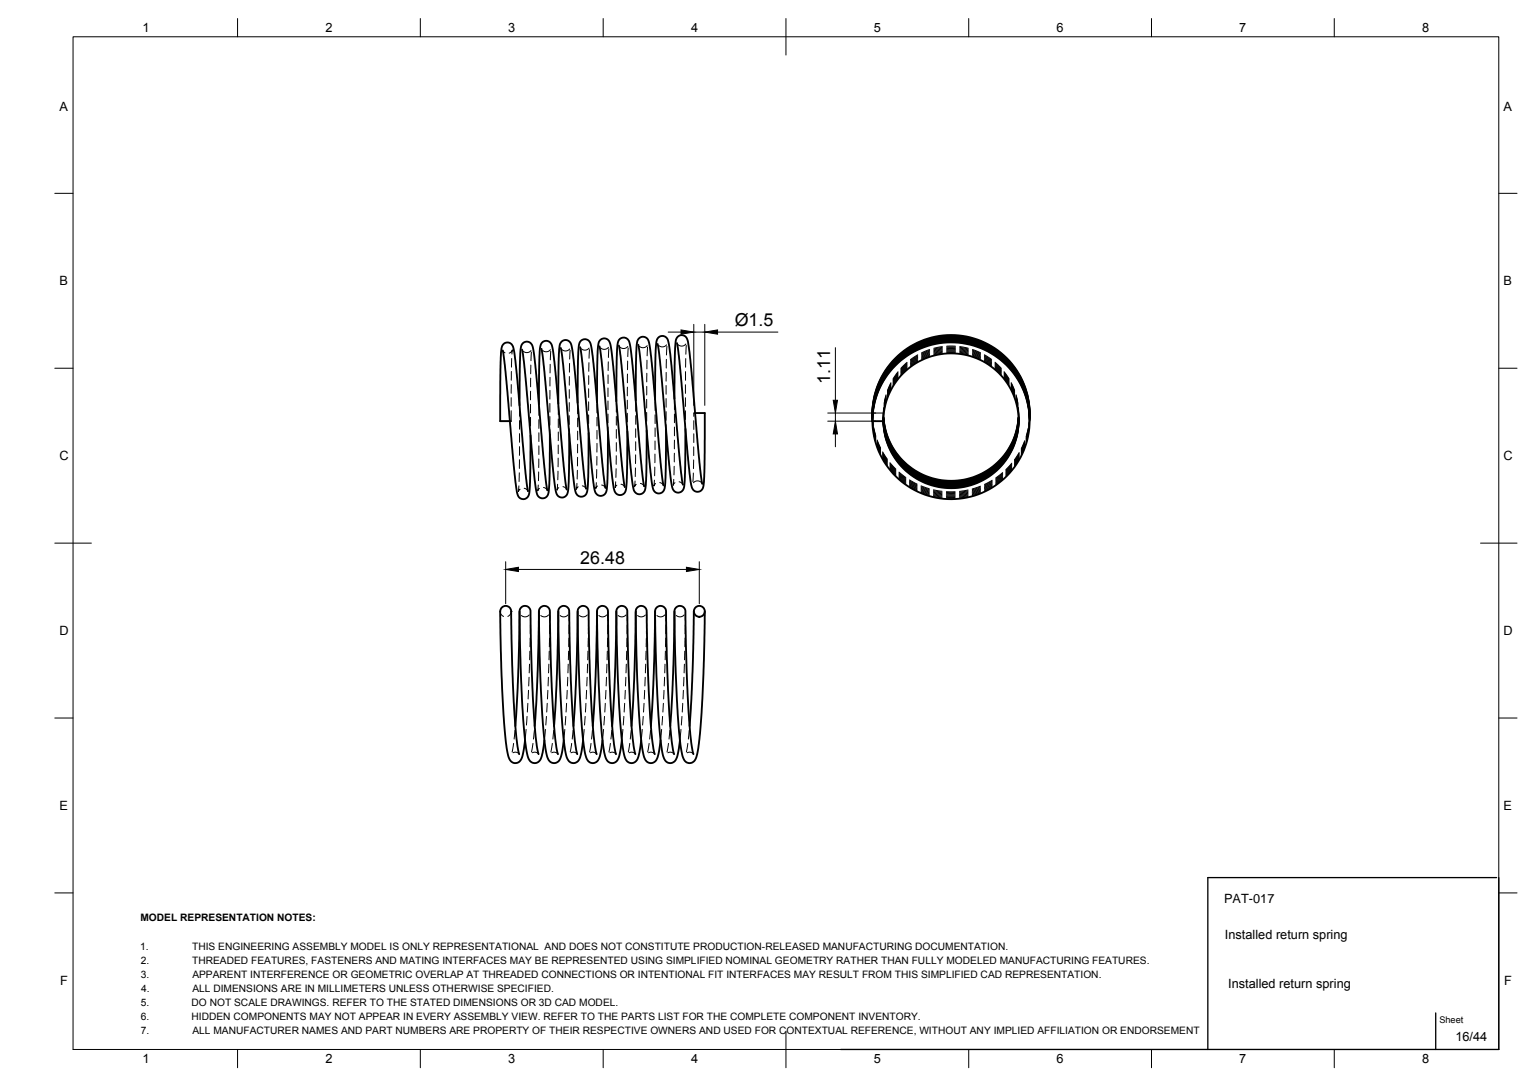
ISO-10303-21;
HEADER;
/* Generated by software containing ST-Developer
 * from STEP Tools, Inc. (www.steptools.com) 
 */

FILE_DESCRIPTION(
/* description */ ('Cam-and-follower valve demonstrator'),
/* implementation_level */ '2;1');

FILE_NAME(
/* name */ 'Installed return spring.step',
/* time_stamp */ '2026-10-28T03:25:17-07:00',
/* author */ (''),
/* organization */ (''),
/* preprocessor_version */ 'ST-DEVELOPER v20.2',
/* originating_system */ 'Autodesk Translation Framework v15.17.0.0',
/* authorisation */ '');

FILE_SCHEMA (('AUTOMOTIVE_DESIGN { 1 0 10303 214 3 1 1 }'));
ENDSEC;

DATA;
#10=MECHANICAL_DESIGN_GEOMETRIC_PRESENTATION_REPRESENTATION('',(#423),#12896);
#324=B_SPLINE_CURVE_WITH_KNOTS('',3,(#11366,#11367,#11368,#11369,#11370,
#11371,#11372,#11373,#11374,#11375,#11376,#11377,#11378,#11379,#11380,#11381,
#11382,#11383,#11384,#11385,#11386,#11387,#11388,#11389,#11390,#11391,#11392,
#11393,#11394,#11395,#11396,#11397,#11398,#11399,#11400,#11401,#11402,#11403,
#11404,#11405,#11406,#11407,#11408,#11409,#11410,#11411,#11412,#11413,#11414,
#11415,#11416,#11417,#11418,#11419,#11420,#11421,#11422,#11423,#11424,#11425,
#11426,#11427,#11428,#11429,#11430,#11431,#11432,#11433,#11434,#11435,#11436,
#11437,#11438,#11439,#11440,#11441,#11442,#11443,#11444,#11445,#11446,#11447,
#11448,#11449,#11450,#11451,#11452,#11453,#11454,#11455,#11456,#11457,#11458,
#11459,#11460,#11461,#11462,#11463,#11464,#11465,#11466,#11467,#11468,#11469,
#11470,#11471,#11472,#11473,#11474,#11475,#11476,#11477,#11478,#11479,#11480,
#11481,#11482,#11483,#11484,#11485,#11486,#11487,#11488,#11489),
 .UNSPECIFIED.,.F.,.F.,(4,1,1,1,1,1,1,1,1,1,1,1,1,1,1,1,1,1,1,1,1,1,1,1,
1,1,1,1,1,1,1,1,1,1,1,1,1,1,1,1,1,1,1,1,1,1,1,1,1,1,1,1,1,1,1,1,1,1,1,1,
1,1,1,1,1,1,1,1,1,1,1,1,1,1,1,1,1,1,1,1,1,1,1,1,1,1,1,1,1,1,1,1,1,1,1,1,
1,1,1,1,1,1,1,1,1,1,1,1,1,1,1,1,1,1,1,1,1,1,1,1,1,4),(0.,0.00892857142857143,
0.0178571428571429,0.0267857142857143,0.0357142857142857,0.0446428571428571,
0.0535714285714286,0.0625,0.0714285714285714,0.0803571428571428,0.0892857142857143,
0.0982142857142857,0.107142857142857,0.116071428571429,0.125,0.133928571428571,
0.142857142857143,0.150793650793651,0.158730158730159,0.166666666666667,
0.174603174603175,0.182539682539683,0.19047619047619,0.202380952380952,
0.214285714285714,0.222222222222222,0.23015873015873,0.238095238095238,
0.244047619047619,0.25,0.255952380952381,0.261904761904762,0.273809523809524,
0.285714285714286,0.297619047619048,0.30952380952381,0.321428571428571,
0.333333333333333,0.341269841269841,0.349206349206349,0.357142857142857,
0.365079365079365,0.373015873015873,0.375,0.376984126984127,0.380952380952381,
0.386904761904762,0.392857142857143,0.404761904761905,0.416666666666667,
0.428571428571429,0.4375,0.446428571428571,0.455357142857143,0.464285714285714,
0.468253968253968,0.476190476190476,0.482142857142857,0.488095238095238,
0.494047619047619,0.5,0.508928571428571,0.517857142857143,0.526785714285714,
0.535714285714286,0.544642857142857,0.553571428571429,0.5625,0.571428571428571,
0.580357142857143,0.589285714285714,0.598214285714286,0.607142857142857,
0.616071428571429,0.625,0.633928571428571,0.642857142857143,0.650793650793651,
0.658730158730159,0.666666666666667,0.672619047619048,0.678571428571428,
0.69047619047619,0.696428571428571,0.702380952380952,0.714285714285714,
0.726190476190476,0.732142857142857,0.738095238095238,0.746031746031746,
0.753968253968254,0.761904761904762,0.76984126984127,0.777777777777778,
0.785714285714286,0.787946428571428,0.790178571428571,0.794642857142857,
0.803571428571428,0.808035714285714,0.8125,0.821428571428571,0.830357142857143,
0.839285714285714,0.848214285714286,0.857142857142857,0.866071428571429,
0.875,0.883928571428571,0.892857142857143,0.901785714285714,0.910714285714286,
0.919642857142857,0.928571428571429,0.9375,0.946428571428571,0.955357142857143,
0.964285714285714,0.973214285714286,0.982142857142857,0.991071428571429,
1.),.UNSPECIFIED.);
#339=B_SPLINE_SURFACE_WITH_KNOTS('',3,3,((#10123,#10124,#10125,#10126,#10127,
#10128,#10129,#10130,#10131,#10132,#10133,#10134,#10135,#10136,#10137,#10138,
#10139,#10140,#10141,#10142,#10143,#10144,#10145,#10146,#10147,#10148,#10149,
#10150,#10151,#10152,#10153,#10154,#10155,#10156,#10157,#10158,#10159,#10160,
#10161,#10162,#10163,#10164,#10165,#10166,#10167,#10168,#10169,#10170,#10171,
#10172,#10173,#10174,#10175,#10176,#10177,#10178,#10179,#10180,#10181,#10182,
#10183,#10184,#10185,#10186,#10187,#10188,#10189,#10190,#10191,#10192,#10193,
#10194,#10195,#10196,#10197,#10198,#10199,#10200,#10201,#10202,#10203,#10204,
#10205,#10206,#10207,#10208,#10209,#10210,#10211,#10212,#10213,#10214,#10215,
#10216,#10217,#10218,#10219,#10220,#10221,#10222,#10223,#10224,#10225,#10226,
#10227,#10228,#10229,#10230,#10231,#10232,#10233,#10234,#10235,#10236,#10237,
#10238,#10239,#10240,#10241,#10242,#10243,#10244,#10245,#10246),(#10247,
#10248,#10249,#10250,#10251,#10252,#10253,#10254,#10255,#10256,#10257,#10258,
#10259,#10260,#10261,#10262,#10263,#10264,#10265,#10266,#10267,#10268,#10269,
#10270,#10271,#10272,#10273,#10274,#10275,#10276,#10277,#10278,#10279,#10280,
#10281,#10282,#10283,#10284,#10285,#10286,#10287,#10288,#10289,#10290,#10291,
#10292,#10293,#10294,#10295,#10296,#10297,#10298,#10299,#10300,#10301,#10302,
#10303,#10304,#10305,#10306,#10307,#10308,#10309,#10310,#10311,#10312,#10313,
#10314,#10315,#10316,#10317,#10318,#10319,#10320,#10321,#10322,#10323,#10324,
#10325,#10326,#10327,#10328,#10329,#10330,#10331,#10332,#10333,#10334,#10335,
#10336,#10337,#10338,#10339,#10340,#10341,#10342,#10343,#10344,#10345,#10346,
#10347,#10348,#10349,#10350,#10351,#10352,#10353,#10354,#10355,#10356,#10357,
#10358,#10359,#10360,#10361,#10362,#10363,#10364,#10365,#10366,#10367,#10368,
#10369,#10370),(#10371,#10372,#10373,#10374,#10375,#10376,#10377,#10378,
#10379,#10380,#10381,#10382,#10383,#10384,#10385,#10386,#10387,#10388,#10389,
#10390,#10391,#10392,#10393,#10394,#10395,#10396,#10397,#10398,#10399,#10400,
#10401,#10402,#10403,#10404,#10405,#10406,#10407,#10408,#10409,#10410,#10411,
#10412,#10413,#10414,#10415,#10416,#10417,#10418,#10419,#10420,#10421,#10422,
#10423,#10424,#10425,#10426,#10427,#10428,#10429,#10430,#10431,#10432,#10433,
#10434,#10435,#10436,#10437,#10438,#10439,#10440,#10441,#10442,#10443,#10444,
#10445,#10446,#10447,#10448,#10449,#10450,#10451,#10452,#10453,#10454,#10455,
#10456,#10457,#10458,#10459,#10460,#10461,#10462,#10463,#10464,#10465,#10466,
#10467,#10468,#10469,#10470,#10471,#10472,#10473,#10474,#10475,#10476,#10477,
#10478,#10479,#10480,#10481,#10482,#10483,#10484,#10485,#10486,#10487,#10488,
#10489,#10490,#10491,#10492,#10493,#10494),(#10495,#10496,#10497,#10498,
#10499,#10500,#10501,#10502,#10503,#10504,#10505,#10506,#10507,#10508,#10509,
#10510,#10511,#10512,#10513,#10514,#10515,#10516,#10517,#10518,#10519,#10520,
#10521,#10522,#10523,#10524,#10525,#10526,#10527,#10528,#10529,#10530,#10531,
#10532,#10533,#10534,#10535,#10536,#10537,#10538,#10539,#10540,#10541,#10542,
#10543,#10544,#10545,#10546,#10547,#10548,#10549,#10550,#10551,#10552,#10553,
#10554,#10555,#10556,#10557,#10558,#10559,#10560,#10561,#10562,#10563,#10564,
#10565,#10566,#10567,#10568,#10569,#10570,#10571,#10572,#10573,#10574,#10575,
#10576,#10577,#10578,#10579,#10580,#10581,#10582,#10583,#10584,#10585,#10586,
#10587,#10588,#10589,#10590,#10591,#10592,#10593,#10594,#10595,#10596,#10597,
#10598,#10599,#10600,#10601,#10602,#10603,#10604,#10605,#10606,#10607,#10608,
#10609,#10610,#10611,#10612,#10613,#10614,#10615,#10616,#10617,#10618),
(#10619,#10620,#10621,#10622,#10623,#10624,#10625,#10626,#10627,#10628,
#10629,#10630,#10631,#10632,#10633,#10634,#10635,#10636,#10637,#10638,#10639,
#10640,#10641,#10642,#10643,#10644,#10645,#10646,#10647,#10648,#10649,#10650,
#10651,#10652,#10653,#10654,#10655,#10656,#10657,#10658,#10659,#10660,#10661,
#10662,#10663,#10664,#10665,#10666,#10667,#10668,#10669,#10670,#10671,#10672,
#10673,#10674,#10675,#10676,#10677,#10678,#10679,#10680,#10681,#10682,#10683,
#10684,#10685,#10686,#10687,#10688,#10689,#10690,#10691,#10692,#10693,#10694,
#10695,#10696,#10697,#10698,#10699,#10700,#10701,#10702,#10703,#10704,#10705,
#10706,#10707,#10708,#10709,#10710,#10711,#10712,#10713,#10714,#10715,#10716,
#10717,#10718,#10719,#10720,#10721,#10722,#10723,#10724,#10725,#10726,#10727,
#10728,#10729,#10730,#10731,#10732,#10733,#10734,#10735,#10736,#10737,#10738,
#10739,#10740,#10741,#10742),(#10743,#10744,#10745,#10746,#10747,#10748,
#10749,#10750,#10751,#10752,#10753,#10754,#10755,#10756,#10757,#10758,#10759,
#10760,#10761,#10762,#10763,#10764,#10765,#10766,#10767,#10768,#10769,#10770,
#10771,#10772,#10773,#10774,#10775,#10776,#10777,#10778,#10779,#10780,#10781,
#10782,#10783,#10784,#10785,#10786,#10787,#10788,#10789,#10790,#10791,#10792,
#10793,#10794,#10795,#10796,#10797,#10798,#10799,#10800,#10801,#10802,#10803,
#10804,#10805,#10806,#10807,#10808,#10809,#10810,#10811,#10812,#10813,#10814,
#10815,#10816,#10817,#10818,#10819,#10820,#10821,#10822,#10823,#10824,#10825,
#10826,#10827,#10828,#10829,#10830,#10831,#10832,#10833,#10834,#10835,#10836,
#10837,#10838,#10839,#10840,#10841,#10842,#10843,#10844,#10845,#10846,#10847,
#10848,#10849,#10850,#10851,#10852,#10853,#10854,#10855,#10856,#10857,#10858,
#10859,#10860,#10861,#10862,#10863,#10864,#10865,#10866),(#10867,#10868,
#10869,#10870,#10871,#10872,#10873,#10874,#10875,#10876,#10877,#10878,#10879,
#10880,#10881,#10882,#10883,#10884,#10885,#10886,#10887,#10888,#10889,#10890,
#10891,#10892,#10893,#10894,#10895,#10896,#10897,#10898,#10899,#10900,#10901,
#10902,#10903,#10904,#10905,#10906,#10907,#10908,#10909,#10910,#10911,#10912,
#10913,#10914,#10915,#10916,#10917,#10918,#10919,#10920,#10921,#10922,#10923,
#10924,#10925,#10926,#10927,#10928,#10929,#10930,#10931,#10932,#10933,#10934,
#10935,#10936,#10937,#10938,#10939,#10940,#10941,#10942,#10943,#10944,#10945,
#10946,#10947,#10948,#10949,#10950,#10951,#10952,#10953,#10954,#10955,#10956,
#10957,#10958,#10959,#10960,#10961,#10962,#10963,#10964,#10965,#10966,#10967,
#10968,#10969,#10970,#10971,#10972,#10973,#10974,#10975,#10976,#10977,#10978,
#10979,#10980,#10981,#10982,#10983,#10984,#10985,#10986,#10987,#10988,#10989,
#10990),(#10991,#10992,#10993,#10994,#10995,#10996,#10997,#10998,#10999,
#11000,#11001,#11002,#11003,#11004,#11005,#11006,#11007,#11008,#11009,#11010,
#11011,#11012,#11013,#11014,#11015,#11016,#11017,#11018,#11019,#11020,#11021,
#11022,#11023,#11024,#11025,#11026,#11027,#11028,#11029,#11030,#11031,#11032,
#11033,#11034,#11035,#11036,#11037,#11038,#11039,#11040,#11041,#11042,#11043,
#11044,#11045,#11046,#11047,#11048,#11049,#11050,#11051,#11052,#11053,#11054,
#11055,#11056,#11057,#11058,#11059,#11060,#11061,#11062,#11063,#11064,#11065,
#11066,#11067,#11068,#11069,#11070,#11071,#11072,#11073,#11074,#11075,#11076,
#11077,#11078,#11079,#11080,#11081,#11082,#11083,#11084,#11085,#11086,#11087,
#11088,#11089,#11090,#11091,#11092,#11093,#11094,#11095,#11096,#11097,#11098,
#11099,#11100,#11101,#11102,#11103,#11104,#11105,#11106,#11107,#11108,#11109,
#11110,#11111,#11112,#11113,#11114),(#11115,#11116,#11117,#11118,#11119,
#11120,#11121,#11122,#11123,#11124,#11125,#11126,#11127,#11128,#11129,#11130,
#11131,#11132,#11133,#11134,#11135,#11136,#11137,#11138,#11139,#11140,#11141,
#11142,#11143,#11144,#11145,#11146,#11147,#11148,#11149,#11150,#11151,#11152,
#11153,#11154,#11155,#11156,#11157,#11158,#11159,#11160,#11161,#11162,#11163,
#11164,#11165,#11166,#11167,#11168,#11169,#11170,#11171,#11172,#11173,#11174,
#11175,#11176,#11177,#11178,#11179,#11180,#11181,#11182,#11183,#11184,#11185,
#11186,#11187,#11188,#11189,#11190,#11191,#11192,#11193,#11194,#11195,#11196,
#11197,#11198,#11199,#11200,#11201,#11202,#11203,#11204,#11205,#11206,#11207,
#11208,#11209,#11210,#11211,#11212,#11213,#11214,#11215,#11216,#11217,#11218,
#11219,#11220,#11221,#11222,#11223,#11224,#11225,#11226,#11227,#11228,#11229,
#11230,#11231,#11232,#11233,#11234,#11235,#11236,#11237,#11238),(#11239,
#11240,#11241,#11242,#11243,#11244,#11245,#11246,#11247,#11248,#11249,#11250,
#11251,#11252,#11253,#11254,#11255,#11256,#11257,#11258,#11259,#11260,#11261,
#11262,#11263,#11264,#11265,#11266,#11267,#11268,#11269,#11270,#11271,#11272,
#11273,#11274,#11275,#11276,#11277,#11278,#11279,#11280,#11281,#11282,#11283,
#11284,#11285,#11286,#11287,#11288,#11289,#11290,#11291,#11292,#11293,#11294,
#11295,#11296,#11297,#11298,#11299,#11300,#11301,#11302,#11303,#11304,#11305,
#11306,#11307,#11308,#11309,#11310,#11311,#11312,#11313,#11314,#11315,#11316,
#11317,#11318,#11319,#11320,#11321,#11322,#11323,#11324,#11325,#11326,#11327,
#11328,#11329,#11330,#11331,#11332,#11333,#11334,#11335,#11336,#11337,#11338,
#11339,#11340,#11341,#11342,#11343,#11344,#11345,#11346,#11347,#11348,#11349,
#11350,#11351,#11352,#11353,#11354,#11355,#11356,#11357,#11358,#11359,#11360,
#11361,#11362)),.UNSPECIFIED.,.T.,.F.,.F.,(4,1,1,1,1,1,1,4),(4,1,1,1,1,
1,1,1,1,1,1,1,1,1,1,1,1,1,1,1,1,1,1,1,1,1,1,1,1,1,1,1,1,1,1,1,1,1,1,1,1,
1,1,1,1,1,1,1,1,1,1,1,1,1,1,1,1,1,1,1,1,1,1,1,1,1,1,1,1,1,1,1,1,1,1,1,1,
1,1,1,1,1,1,1,1,1,1,1,1,1,1,1,1,1,1,1,1,1,1,1,1,1,1,1,1,1,1,1,1,1,1,1,1,
1,1,1,1,1,1,1,1,4),(-3.14159265358979,-2.24399475256414,-1.34639685153848,
-0.448798950512828,0.448798950512828,1.34639685153848,2.24399475256414,
3.14159265358979),(0.,0.00892857142857143,0.0178571428571429,0.0267857142857143,
0.0357142857142857,0.0446428571428571,0.0535714285714286,0.0625,0.0714285714285714,
0.0803571428571428,0.0892857142857143,0.0982142857142857,0.107142857142857,
0.116071428571429,0.125,0.133928571428571,0.142857142857143,0.150793650793651,
0.158730158730159,0.166666666666667,0.174603174603175,0.182539682539683,
0.19047619047619,0.202380952380952,0.214285714285714,0.222222222222222,
0.23015873015873,0.238095238095238,0.244047619047619,0.25,0.255952380952381,
0.261904761904762,0.273809523809524,0.285714285714286,0.297619047619048,
0.30952380952381,0.321428571428571,0.333333333333333,0.341269841269841,
0.349206349206349,0.357142857142857,0.365079365079365,0.373015873015873,
0.375,0.376984126984127,0.380952380952381,0.386904761904762,0.392857142857143,
0.404761904761905,0.416666666666667,0.428571428571429,0.4375,0.446428571428571,
0.455357142857143,0.464285714285714,0.468253968253968,0.476190476190476,
0.482142857142857,0.488095238095238,0.494047619047619,0.5,0.508928571428571,
0.517857142857143,0.526785714285714,0.535714285714286,0.544642857142857,
0.553571428571429,0.5625,0.571428571428571,0.580357142857143,0.589285714285714,
0.598214285714286,0.607142857142857,0.616071428571429,0.625,0.633928571428571,
0.642857142857143,0.650793650793651,0.658730158730159,0.666666666666667,
0.672619047619048,0.678571428571428,0.69047619047619,0.696428571428571,
0.702380952380952,0.714285714285714,0.726190476190476,0.732142857142857,
0.738095238095238,0.746031746031746,0.753968253968254,0.761904761904762,
0.76984126984127,0.777777777777778,0.785714285714286,0.787946428571428,
0.790178571428571,0.794642857142857,0.803571428571428,0.808035714285714,
0.8125,0.821428571428571,0.830357142857143,0.839285714285714,0.848214285714286,
0.857142857142857,0.866071428571429,0.875,0.883928571428571,0.892857142857143,
0.901785714285714,0.910714285714286,0.919642857142857,0.928571428571429,
0.9375,0.946428571428571,0.955357142857143,0.964285714285714,0.973214285714286,
0.982142857142857,0.991071428571429,1.),.UNSPECIFIED.);
#351=SHAPE_REPRESENTATION_RELATIONSHIP('SRR','None',#13067,#387);
#387=ADVANCED_BREP_SHAPE_REPRESENTATION('',(#466),#12867);
#423=STYLED_ITEM('',(#13330),#466);
#466=MANIFOLD_SOLID_BREP('Body1',#6190);
#789=CIRCLE('',#6910,0.075);
#790=CIRCLE('',#6911,0.075);
#1239=FACE_OUTER_BOUND('',#1716,.T.);
#1240=FACE_OUTER_BOUND('',#1717,.T.);
#1241=FACE_OUTER_BOUND('',#1718,.T.);
#1716=EDGE_LOOP('',(#4749,#4750,#4751,#4752));
#1717=EDGE_LOOP('',(#4753));
#1718=EDGE_LOOP('',(#4754));
#3057=VERTEX_POINT('',#11363);
#3058=VERTEX_POINT('',#11365);
#3671=EDGE_CURVE('',#3057,#3057,#789,.T.);
#3672=EDGE_CURVE('',#3057,#3058,#324,.T.);
#3673=EDGE_CURVE('',#3058,#3058,#790,.T.);
#4749=ORIENTED_EDGE('',*,*,#3671,.T.);
#4750=ORIENTED_EDGE('',*,*,#3672,.T.);
#4751=ORIENTED_EDGE('',*,*,#3673,.F.);
#4752=ORIENTED_EDGE('',*,*,#3672,.F.);
#4753=ORIENTED_EDGE('',*,*,#3673,.T.);
#4754=ORIENTED_EDGE('',*,*,#3671,.F.);
#5676=PLANE('',#6912);
#5677=PLANE('',#6913);
#5955=ADVANCED_FACE('',(#1239),#339,.T.);
#5956=ADVANCED_FACE('',(#1240),#5676,.T.);
#5957=ADVANCED_FACE('',(#1241),#5677,.F.);
#6190=CLOSED_SHELL('',(#5955,#5956,#5957));
#6909=AXIS2_PLACEMENT_3D('',#10122,#8185,#8186);
#6910=AXIS2_PLACEMENT_3D('',#11364,#8187,#8188);
#6911=AXIS2_PLACEMENT_3D('',#11490,#8189,#8190);
#6912=AXIS2_PLACEMENT_3D('',#11491,#8191,#8192);
#6913=AXIS2_PLACEMENT_3D('',#11492,#8193,#8194);
#8185=DIRECTION('axis',(0.,0.,1.));
#8186=DIRECTION('refdir',(1.,0.,0.));
#8187=DIRECTION('center_axis',(-0.00013450227597807,0.999117050244768,0.042013114849203));
#8188=DIRECTION('ref_axis',(5.65585335115278E-6,-0.0420131144685042,0.999117059298192));
#8189=DIRECTION('center_axis',(0.000134502259908405,0.999117050228794,0.0420131152291186));
#8190=DIRECTION('ref_axis',(-0.474109261639291,0.0370548329511252,-0.879685936788131));
#8191=DIRECTION('center_axis',(0.000134502259908405,0.999117050228794,0.0420131152291186));
#8192=DIRECTION('ref_axis',(-0.474109261639291,0.0370548329511252,-0.879685936788131));
#8193=DIRECTION('center_axis',(-0.00013450227597807,0.999117050244768,0.042013114849203));
#8194=DIRECTION('ref_axis',(5.65585335115278E-6,-0.0420131144685042,0.999117059298193));
#10122=CARTESIAN_POINT('',(0.,0.,0.));
#10123=CARTESIAN_POINT('Ctrl Pts',(0.999999575810999,0.00315098358513781,
7.20006622055264));
#10124=CARTESIAN_POINT('Ctrl Pts',(0.999974319608277,0.190760468856422,
7.20795524501636));
#10125=CARTESIAN_POINT('Ctrl Pts',(0.892344234443071,0.564401735476683,
7.22374165130483));
#10126=CARTESIAN_POINT('Ctrl Pts',(0.456170863303355,0.954569139239392,
7.24746551842362));
#10127=CARTESIAN_POINT('Ctrl Pts',(-0.121643296695006,1.0527111229517,7.27123039275792));
#10128=CARTESIAN_POINT('Ctrl Pts',(-0.664174499114347,0.828146653873478,
7.29503750827097));
#10129=CARTESIAN_POINT('Ctrl Pts',(-1.00466229107333,0.348451955041142,
7.31888617441183));
#10130=CARTESIAN_POINT('Ctrl Pts',(-1.03783821085617,-0.239862803165599,
7.34277653444097));
#10131=CARTESIAN_POINT('Ctrl Pts',(-0.752436914310739,-0.756562482852077,
7.36670833282365));
#10132=CARTESIAN_POINT('Ctrl Pts',(-0.234997931414651,-1.04270891419437,
7.39068146490982));
#10133=CARTESIAN_POINT('Ctrl Pts',(0.356377432582172,-1.00964746384867,
7.41469572763747));
#10134=CARTESIAN_POINT('Ctrl Pts',(0.840341677037224,-0.666437865062604,
7.43875093208249));
#10135=CARTESIAN_POINT('Ctrl Pts',(1.06790358406505,-0.117422164195028,
7.4628468515188));
#10136=CARTESIAN_POINT('Ctrl Pts',(0.968336509361683,0.469494166098508,
7.48698324256581));
#10137=CARTESIAN_POINT('Ctrl Pts',(0.571081336399399,0.914217869413367,
7.51115983904362));
#10138=CARTESIAN_POINT('Ctrl Pts',(-0.00276942901145937,1.07968430615977,
7.53537635143244));
#10139=CARTESIAN_POINT('Ctrl Pts',(-0.577781503135752,0.914223804149117,
7.55963247041146));
#10140=CARTESIAN_POINT('Ctrl Pts',(-0.962145622562424,0.483976677731404,
7.58302803095162));
#10141=CARTESIAN_POINT('Ctrl Pts',(-1.07125753086067,-0.0562794445165808,
7.60555779623404));
#10142=CARTESIAN_POINT('Ctrl Pts',(-0.915194862614763,-0.562561634031091,
7.6272168563822));
#10143=CARTESIAN_POINT('Ctrl Pts',(-0.53551487530705,-0.932963762094015,
7.64890612590553));
#10144=CARTESIAN_POINT('Ctrl Pts',(-0.024035065806305,-1.07736876663697,
7.67062531437742));
#10145=CARTESIAN_POINT('Ctrl Pts',(0.494146757015346,-0.958466814289234,
7.69237411680017));
#10146=CARTESIAN_POINT('Ctrl Pts',(0.961479539986573,-0.548279772601945,
7.71778190065853));
#10147=CARTESIAN_POINT('Ctrl Pts',(1.12756301652098,0.172482400610549,7.74686765103336));
#10148=CARTESIAN_POINT('Ctrl Pts',(0.75611713355168,0.813684959589575,7.77601030696451));
#10149=CARTESIAN_POINT('Ctrl Pts',(0.185875815215743,1.06965010757807,7.80155082448588));
#10150=CARTESIAN_POINT('Ctrl Pts',(-0.348517058347165,1.02984652160674,
7.82347022110603));
#10151=CARTESIAN_POINT('Ctrl Pts',(-0.761949296282463,0.762592777124389,
7.84358787235736));
#10152=CARTESIAN_POINT('Ctrl Pts',(-0.996722963062006,0.388518849169714,
7.86189613571743));
#10153=CARTESIAN_POINT('Ctrl Pts',(-1.07098690831041,-0.00260829917091459,
7.87838843437341));
#10154=CARTESIAN_POINT('Ctrl Pts',(-0.99661183226746,-0.393594984460838,
7.894895410549));
#10155=CARTESIAN_POINT('Ctrl Pts',(-0.714908576434247,-0.844892296878379,
7.9169240469514));
#10156=CARTESIAN_POINT('Ctrl Pts',(-0.084422651145012,-1.14985023564212,
7.94449562780488));
#10157=CARTESIAN_POINT('Ctrl Pts',(0.721887320494981,-0.901498071462995,
7.97763725360595));
#10158=CARTESIAN_POINT('Ctrl Pts',(1.14390600676876,-0.170383526932712,
8.01083302661308));
#10159=CARTESIAN_POINT('Ctrl Pts',(0.956311918053777,0.65401391794098,8.04408130906187));
#10160=CARTESIAN_POINT('Ctrl Pts',(0.25602906697655,1.13176193513965,8.07738040653961));
#10161=CARTESIAN_POINT('Ctrl Pts',(-0.488510543500641,1.01860423556296,
8.10702323570327));
#10162=CARTESIAN_POINT('Ctrl Pts',(-0.942716248260153,0.573655629467007,
8.13299136011509));
#10163=CARTESIAN_POINT('Ctrl Pts',(-1.10358636285334,0.0534364176198665,
8.15527022722507));
#10164=CARTESIAN_POINT('Ctrl Pts',(-0.99543872479676,-0.481361877750802,
8.17756901902506));
#10165=CARTESIAN_POINT('Ctrl Pts',(-0.644826641417894,-0.899786909633448,
8.1998871769012));
#10166=CARTESIAN_POINT('Ctrl Pts',(-0.263312902512338,-1.04918995788175,
8.21663989380025));
#10167=CARTESIAN_POINT('Ctrl Pts',(0.00166665731618679,-1.0655343402046,
8.22781406534667));
#10168=CARTESIAN_POINT('Ctrl Pts',(0.178270288589001,-1.05454413855026,
8.23526501957515));
#10169=CARTESIAN_POINT('Ctrl Pts',(0.437439999691742,-0.98876491629653,
8.24644481283225));
#10170=CARTESIAN_POINT('Ctrl Pts',(0.741357296669408,-0.797196125183601,
8.26135855011107));
#10171=CARTESIAN_POINT('Ctrl Pts',(1.06427742047819,-0.363196133741635,
8.28374205636937));
#10172=CARTESIAN_POINT('Ctrl Pts',(1.1191132547847,0.345488423812591,8.31174498186711));
#10173=CARTESIAN_POINT('Ctrl Pts',(0.584140656179565,1.01596202851522,8.34538413710338));
#10174=CARTESIAN_POINT('Ctrl Pts',(-0.19096844855633,1.13165287559935,8.37625078730322));
#10175=CARTESIAN_POINT('Ctrl Pts',(-0.797411359462935,0.795301993540907,
8.40433431031039));
#10176=CARTESIAN_POINT('Ctrl Pts',(-1.0990783559073,0.250015446968417,8.4296262708737));
#10177=CARTESIAN_POINT('Ctrl Pts',(-1.06426569125542,-0.373802040240765,
8.45493410201599));
#10178=CARTESIAN_POINT('Ctrl Pts',(-0.769553388901587,-0.788092512102153,
8.47556748693345));
#10179=CARTESIAN_POINT('Ctrl Pts',(-0.367608264833719,-1.03377453912702,
8.49527086803642));
#10180=CARTESIAN_POINT('Ctrl Pts',(0.0389894662197936,-1.10568483145998,
8.51216552927169));
#10181=CARTESIAN_POINT('Ctrl Pts',(0.476842798425807,-0.987859734068039,
8.53094473644388));
#10182=CARTESIAN_POINT('Ctrl Pts',(0.805101130351003,-0.7459169684144,8.54785141982868));
#10183=CARTESIAN_POINT('Ctrl Pts',(1.02206224073455,-0.400294829517718,
8.56476322077897));
#10184=CARTESIAN_POINT('Ctrl Pts',(1.11108597940432,0.0676090739442989,
8.58449929513004));
#10185=CARTESIAN_POINT('Ctrl Pts',(0.957486327179168,0.602305552598091,
8.60706239241156));
#10186=CARTESIAN_POINT('Ctrl Pts',(0.490319176226327,1.0196961225561,8.63245514939238));
#10187=CARTESIAN_POINT('Ctrl Pts',(-0.127227772869885,1.12465246691674,
8.65785621578684));
#10188=CARTESIAN_POINT('Ctrl Pts',(-0.706252354762176,0.884861784560879,
8.6832646175365));
#10189=CARTESIAN_POINT('Ctrl Pts',(-1.06898139570907,0.373646110671472,
8.70867937640931));
#10190=CARTESIAN_POINT('Ctrl Pts',(-1.10415883703196,-0.252336062683339,
8.73409951326223));
#10191=CARTESIAN_POINT('Ctrl Pts',(-0.800834752831557,-0.801177522527246,
8.75952404569165));
#10192=CARTESIAN_POINT('Ctrl Pts',(-0.251930241323733,-1.10455619700772,
8.78495198825788));
#10193=CARTESIAN_POINT('Ctrl Pts',(0.374309533721303,-1.06939244573458,
8.81038235029736));
#10194=CARTESIAN_POINT('Ctrl Pts',(0.88588373813812,-0.706416051605379,
8.83581414648952));
#10195=CARTESIAN_POINT('Ctrl Pts',(1.12593002076033,-0.126889341474946,
8.86124638643539));
#10196=CARTESIAN_POINT('Ctrl Pts',(1.02087104515559,0.491507891337351,8.88667807898767));
#10197=CARTESIAN_POINT('Ctrl Pts',(0.602911335681679,0.959196578831539,
8.91210823370906));
#10198=CARTESIAN_POINT('Ctrl Pts',(0.000316973456126708,1.13280882473463,
8.93753586563178));
#10199=CARTESIAN_POINT('Ctrl Pts',(-0.602311983560242,0.959240722445107,
8.9629599838141));
#10200=CARTESIAN_POINT('Ctrl Pts',(-1.00436822137552,0.509038661422071,
8.98743813657581));
#10201=CARTESIAN_POINT('Ctrl Pts',(-1.11811011681427,-0.0552669144060651,
9.01097002817133));
#10202=CARTESIAN_POINT('Ctrl Pts',(-0.955644771077333,-0.583087731975911,
9.03355562561233));
#10203=CARTESIAN_POINT('Ctrl Pts',(-0.593074356957321,-0.936728146430118,
9.0542538609391));
#10204=CARTESIAN_POINT('Ctrl Pts',(-0.164731041598437,-1.08578943530602,
9.07306578079699));
#10205=CARTESIAN_POINT('Ctrl Pts',(0.380219776536112,-1.06693040182505,
9.09563491033651));
#10206=CARTESIAN_POINT('Ctrl Pts',(0.853779549938941,-0.745621203287222,
9.11819570154211));
#10207=CARTESIAN_POINT('Ctrl Pts',(1.06953462325323,-0.245092836305948,
9.14074702398398));
#10208=CARTESIAN_POINT('Ctrl Pts',(1.09185195352203,0.298202592837182,9.16329164905568));
#10209=CARTESIAN_POINT('Ctrl Pts',(0.734297058725123,0.919425032182445,
9.19145918094331));
#10210=CARTESIAN_POINT('Ctrl Pts',(0.0501860572080287,1.12913650428628,
9.21960716991184));
#10211=CARTESIAN_POINT('Ctrl Pts',(-0.47422284767955,0.986938013732599,
9.24211273100823));
#10212=CARTESIAN_POINT('Ctrl Pts',(-0.83834294439581,0.718994011703782,
9.26085993499593));
#10213=CARTESIAN_POINT('Ctrl Pts',(-1.0797140885543,0.276058653254629,9.28147192866405));
#10214=CARTESIAN_POINT('Ctrl Pts',(-1.0792869722179,-0.273490761429736,
9.30394472055128));
#10215=CARTESIAN_POINT('Ctrl Pts',(-0.816874083948392,-0.756154521252702,
9.32640385818033));
#10216=CARTESIAN_POINT('Ctrl Pts',(-0.355458797527567,-1.05362205517351,
9.34884870640624));
#10217=CARTESIAN_POINT('Ctrl Pts',(0.191577194376755,-1.09493860698716,
9.37127864639074));
#10218=CARTESIAN_POINT('Ctrl Pts',(0.571484722667441,-0.923210767165354,
9.38832293897591));
#10219=CARTESIAN_POINT('Ctrl Pts',(0.775578610165073,-0.735373724461368,
9.39999172743641));
#10220=CARTESIAN_POINT('Ctrl Pts',(0.90219668945127,-0.581077610283799,
9.40839153478326));
#10221=CARTESIAN_POINT('Ctrl Pts',(1.06423218001646,-0.268505675241936,
9.42308663622534));
#10222=CARTESIAN_POINT('Ctrl Pts',(1.08737574685665,0.14445700622961,9.43987039483926));
#10223=CARTESIAN_POINT('Ctrl Pts',(0.943512119332504,0.519555849049532,
9.45664308969273));
#10224=CARTESIAN_POINT('Ctrl Pts',(0.702595952885493,0.840663912121189,
9.47340826939813));
#10225=CARTESIAN_POINT('Ctrl Pts',(0.250731034525726,1.09066378632527,9.49435038976507));
#10226=CARTESIAN_POINT('Ctrl Pts',(-0.367646366337481,1.05577469318307,
9.51945715090945));
#10227=CARTESIAN_POINT('Ctrl Pts',(-0.872073427555176,0.697769149747224,
9.54453931621249));
#10228=CARTESIAN_POINT('Ctrl Pts',(-1.10851395153864,0.126754498956172,
9.56959609551394));
#10229=CARTESIAN_POINT('Ctrl Pts',(-1.004997965557,-0.481859237919703,9.59462670660628));
#10230=CARTESIAN_POINT('Ctrl Pts',(-0.593994937248818,-0.94163509404227,
9.61963038098806));
#10231=CARTESIAN_POINT('Ctrl Pts',(-0.0020235655980388,-1.11207375119343,
9.6446063758667));
#10232=CARTESIAN_POINT('Ctrl Pts',(0.589215999041395,-0.941636436533483,
9.66955394755264));
#10233=CARTESIAN_POINT('Ctrl Pts',(0.99867475328867,-0.483298149068583,
9.69447238340543));
#10234=CARTESIAN_POINT('Ctrl Pts',(1.10139617547556,0.121906639873499,9.71936097538517));
#10235=CARTESIAN_POINT('Ctrl Pts',(0.866669607038716,0.688301956936916,
9.74421904187644));
#10236=CARTESIAN_POINT('Ctrl Pts',(0.367204775824758,1.0425526426198,9.76904590972932));
#10237=CARTESIAN_POINT('Ctrl Pts',(-0.243395435261487,1.07672488055471,
9.79384092765142));
#10238=CARTESIAN_POINT('Ctrl Pts',(-0.777888567237211,0.781186417289152,
9.81860345995005));
#10239=CARTESIAN_POINT('Ctrl Pts',(-1.07283036518199,0.247282943918733,
9.84333289822209));
#10240=CARTESIAN_POINT('Ctrl Pts',(-1.03856704754786,-0.360866232625645,
9.86802861303319));
#10241=CARTESIAN_POINT('Ctrl Pts',(-0.686501281653619,-0.856920605922548,
9.892690097101));
#10242=CARTESIAN_POINT('Ctrl Pts',(-0.125304938207573,-1.08924443021579,
9.91731661435472));
#10243=CARTESIAN_POINT('Ctrl Pts',(0.472593334675849,-0.987703022851267,
9.94190800522239));
#10244=CARTESIAN_POINT('Ctrl Pts',(0.924078607982629,-0.583894056083662,
9.9664628819065));
#10245=CARTESIAN_POINT('Ctrl Pts',(1.03553205098759,-0.196980695813872,
9.98281022139497));
#10246=CARTESIAN_POINT('Ctrl Pts',(1.03555819462295,-0.00277911247133682,
9.99097644525911));
#10247=CARTESIAN_POINT('Ctrl Pts',(0.977559628488695,0.00314796269385491,
7.20006622055264));
#10248=CARTESIAN_POINT('Ctrl Pts',(0.977534931919559,0.186600347624405,
7.20778043793643));
#10249=CARTESIAN_POINT('Ctrl Pts',(0.872326621716519,0.551848843788545,
7.22321134603222));
#10250=CARTESIAN_POINT('Ctrl Pts',(0.445888516650333,0.933334827963534,
7.24640607517782));
#10251=CARTESIAN_POINT('Ctrl Pts',(-0.119073548305639,1.02929389999416,
7.26964128868359));
#10252=CARTESIAN_POINT('Ctrl Pts',(-0.649587147996202,0.80971547210797,
7.29292023194622));
#10253=CARTESIAN_POINT('Ctrl Pts',(-0.982569682264781,0.340608289962485,
7.31624170699604));
#10254=CARTESIAN_POINT('Ctrl Pts',(-1.01502761301115,-0.234786092628464,
7.33960648723202));
#10255=CARTESIAN_POINT('Ctrl Pts',(-0.735871175247769,-0.740204838677808,
7.36301444474564));
#10256=CARTESIAN_POINT('Ctrl Pts',(-0.229676322236327,-1.02014816093488,
7.3864658304475));
#10257=CARTESIAN_POINT('Ctrl Pts',(0.348937939981405,-0.987814457701798,
7.4099606987694));
#10258=CARTESIAN_POINT('Ctrl Pts',(0.822539330220122,-0.651972394453966,
7.43349915759815));
#10259=CARTESIAN_POINT('Ctrl Pts',(1.04527595941213,-0.114640290127698,
7.45708126355647));
#10260=CARTESIAN_POINT('Ctrl Pts',(0.947826468806296,0.459896400546727,
7.48070704898826));
#10261=CARTESIAN_POINT('Ctrl Pts',(0.55889347637454,0.895331088517642,7.50437654814852));
#10262=CARTESIAN_POINT('Ctrl Pts',(-0.00306079128538847,1.05738788811831,
7.52808969478327));
#10263=CARTESIAN_POINT('Ctrl Pts',(-0.566280527706047,0.895342454830755,
7.55184656451516));
#10264=CARTESIAN_POINT('Ctrl Pts',(-0.94285566098478,0.473846121224849,
7.57476532068617));
#10265=CARTESIAN_POINT('Ctrl Pts',(-1.0497916614659,-0.0555531181652621,
7.59684113555968));
#10266=CARTESIAN_POINT('Ctrl Pts',(-0.896848267782611,-0.551773383072111,
7.6180679179377));
#10267=CARTESIAN_POINT('Ctrl Pts',(-0.524644889084921,-0.914897925677014,
7.63932924215096));
#10268=CARTESIAN_POINT('Ctrl Pts',(-0.0231086211666074,-1.0565167949332,
7.66062527908679));
#10269=CARTESIAN_POINT('Ctrl Pts',(0.485127965286644,-0.939908247511382,
7.6819553795526));
#10270=CARTESIAN_POINT('Ctrl Pts',(0.943615377154503,-0.537522345290259,
7.70687961457021));
#10271=CARTESIAN_POINT('Ctrl Pts',(1.10664549720515,0.169763989700331,7.73541865071932));
#10272=CARTESIAN_POINT('Ctrl Pts',(0.742051547502606,0.79926014258511,7.76402418077492));
#10273=CARTESIAN_POINT('Ctrl Pts',(0.1820386242008,1.05066099789059,7.78910535841451));
#10274=CARTESIAN_POINT('Ctrl Pts',(-0.342925213792071,1.01157659627672,
7.81063708262925));
#10275=CARTESIAN_POINT('Ctrl Pts',(-0.749174696900719,0.748993162117811,
7.83040267717073));
#10276=CARTESIAN_POINT('Ctrl Pts',(-0.979935807647696,0.381329024216996,
7.84839633933116));
#10277=CARTESIAN_POINT('Ctrl Pts',(-1.05295127075641,-0.0031834724715258,
7.86460871683656));
#10278=CARTESIAN_POINT('Ctrl Pts',(-0.979823859029814,-0.387650529628831,
7.88083924305493));
#10279=CARTESIAN_POINT('Ctrl Pts',(-0.702763365403678,-0.831532214326253,
7.9025045281952));
#10280=CARTESIAN_POINT('Ctrl Pts',(-0.0824799953521556,-1.13161645631995,
7.92962705663339));
#10281=CARTESIAN_POINT('Ctrl Pts',(0.711242926121418,-0.887223370319477,
7.9622469399467));
#10282=CARTESIAN_POINT('Ctrl Pts',(1.12693381986534,-0.167219554477753,
7.99493570676171));
#10283=CARTESIAN_POINT('Ctrl Pts',(0.942170158410588,0.645122540676551,
8.02769289174508));
#10284=CARTESIAN_POINT('Ctrl Pts',(0.251833448908431,1.11619302546554,8.06051740773355));
#10285=CARTESIAN_POINT('Ctrl Pts',(-0.482576734552971,1.00466065240982,
8.08975175083041));
#10286=CARTESIAN_POINT('Ctrl Pts',(-0.930837186086348,0.565588449238039,
8.1153761207135));
#10287=CARTESIAN_POINT('Ctrl Pts',(-1.08967697962172,0.0520404847636478,
8.13736727171514));
#10288=CARTESIAN_POINT('Ctrl Pts',(-0.982903963949899,-0.476104949614679,
8.15938616711863));
#10289=CARTESIAN_POINT('Ctrl Pts',(-0.636540954845654,-0.889508172876264,
8.18143408833578));
#10290=CARTESIAN_POINT('Ctrl Pts',(-0.259505287977444,-1.03717085636039,
8.1979881155864));
#10291=CARTESIAN_POINT('Ctrl Pts',(0.00245412741644389,-1.05333143683712,
8.20903477211785));
#10292=CARTESIAN_POINT('Ctrl Pts',(0.177059177795229,-1.04246573347879,
8.21640112872543));
#10293=CARTESIAN_POINT('Ctrl Pts',(0.433327913156591,-0.977427600945312,
8.22745510314132));
#10294=CARTESIAN_POINT('Ctrl Pts',(0.73391120866048,-0.78797120607176,8.2422033360845));
#10295=CARTESIAN_POINT('Ctrl Pts',(1.05339268942341,-0.358614771787532,
8.26434632322957));
#10296=CARTESIAN_POINT('Ctrl Pts',(1.10774289737246,0.342815554655969,8.29206074311086));
#10297=CARTESIAN_POINT('Ctrl Pts',(0.578013407396415,1.00685700818336,8.32536809202379));
#10298=CARTESIAN_POINT('Ctrl Pts',(-0.190065697378914,1.12158925721513,
8.35595007218663));
#10299=CARTESIAN_POINT('Ctrl Pts',(-0.791379955781598,0.788136209353913,
8.38379141767993));
#10300=CARTESIAN_POINT('Ctrl Pts',(-1.09065818214293,0.247264712325509,
8.40887610904288));
#10301=CARTESIAN_POINT('Ctrl Pts',(-1.05615602025911,-0.371820083200091,
8.43398889502081));
#10302=CARTESIAN_POINT('Ctrl Pts',(-0.763582331280387,-0.783164528531196,
8.45447107190819));
#10303=CARTESIAN_POINT('Ctrl Pts',(-0.364356836371496,-1.02719384800769,
8.47404015218794));
#10304=CARTESIAN_POINT('Ctrl Pts',(0.0396184639487176,-1.0986608375699,
8.49082507049449));
#10305=CARTESIAN_POINT('Ctrl Pts',(0.4747993472484,-0.981570587611574,8.5094874174984));
#10306=CARTESIAN_POINT('Ctrl Pts',(0.801179445412529,-0.741029716701455,
8.52629619867346));
#10307=CARTESIAN_POINT('Ctrl Pts',(1.01695965272321,-0.397307355171047,
8.54311315644057));
#10308=CARTESIAN_POINT('Ctrl Pts',(1.10554233979669,0.0681936417011055,
8.56274660530892));
#10309=CARTESIAN_POINT('Ctrl Pts',(0.952705524054136,0.600346322280504,
8.5851983552402));
#10310=CARTESIAN_POINT('Ctrl Pts',(0.487557651772792,1.01598809297735,8.61047974857097));
#10311=CARTESIAN_POINT('Ctrl Pts',(-0.127651652476803,1.12058418421206,
8.63578130248315));
#10312=CARTESIAN_POINT('Ctrl Pts',(-0.70478866362112,0.881619626848855,
8.66110291473919));
#10313=CARTESIAN_POINT('Ctrl Pts',(-1.06653738915564,0.371858090305246,
8.68644322194209));
#10314=CARTESIAN_POINT('Ctrl Pts',(-1.10167663567818,-0.252676170428594,
8.71180143479237));
#10315=CARTESIAN_POINT('Ctrl Pts',(-0.798942597498512,-0.800540151616223,
8.73717650800646));
#10316=CARTESIAN_POINT('Ctrl Pts',(-0.25078864090532,-1.10355366139075,
8.76256750487144));
#10317=CARTESIAN_POINT('Ctrl Pts',(0.374929053613694,-1.0684625769043,8.7879734299407));
#10318=CARTESIAN_POINT('Ctrl Pts',(0.886351621064952,-0.705646605063887,
8.81339330544931));
#10319=CARTESIAN_POINT('Ctrl Pts',(1.12647324119551,-0.126050893654806,
8.83882613969898));
#10320=CARTESIAN_POINT('Ctrl Pts',(1.02139014639355,0.492749598489448,8.86427091353165));
#10321=CARTESIAN_POINT('Ctrl Pts',(0.602990734075153,0.960997323753939,
8.88972664071518));
#10322=CARTESIAN_POINT('Ctrl Pts',(-0.000567847562754408,1.13493523731139,
8.91519221987827));
#10323=CARTESIAN_POINT('Ctrl Pts',(-0.604479916359356,0.9610454826922,8.94066675637306));
#10324=CARTESIAN_POINT('Ctrl Pts',(-1.00761036182794,0.5097064617892,8.96520501612694));
#10325=CARTESIAN_POINT('Ctrl Pts',(-1.12172878107286,-0.0563180902115076,
8.98880606838067));
#10326=CARTESIAN_POINT('Ctrl Pts',(-0.958723063179525,-0.586004022927428,
9.01146964038096));
#10327=CARTESIAN_POINT('Ctrl Pts',(-0.59474503181829,-0.941054468652076,
9.03224747251221));
#10328=CARTESIAN_POINT('Ctrl Pts',(-0.164564414600358,-1.09076932470309,
9.05113813987772));
#10329=CARTESIAN_POINT('Ctrl Pts',(0.382914792126433,-1.0718353554875,9.07381083702006));
#10330=CARTESIAN_POINT('Ctrl Pts',(0.858914210761414,-0.7489475446806,9.09648289188614));
#10331=CARTESIAN_POINT('Ctrl Pts',(1.07589051190367,-0.245617047231296,
9.1191583368655));
#10332=CARTESIAN_POINT('Ctrl Pts',(1.09835720626968,0.300895372898752,9.14183499997529));
#10333=CARTESIAN_POINT('Ctrl Pts',(0.738597876638515,0.926101901793705,
9.1701764747506));
#10334=CARTESIAN_POINT('Ctrl Pts',(0.0497353559870152,1.13736148182463,
9.19851634662638));
#10335=CARTESIAN_POINT('Ctrl Pts',(-0.478615212533917,0.994112255401606,
9.22118869187345));
#10336=CARTESIAN_POINT('Ctrl Pts',(-0.845581735917551,0.72408762970704,
9.24008098535963));
#10337=CARTESIAN_POINT('Ctrl Pts',(-1.08894413293595,0.27757420396775,9.26085707574209));
#10338=CARTESIAN_POINT('Ctrl Pts',(-1.08853511612709,-0.276687817589094,
9.28352144802081));
#10339=CARTESIAN_POINT('Ctrl Pts',(-0.823804291843437,-0.763690543375918,
9.30617985595382));
#10340=CARTESIAN_POINT('Ctrl Pts',(-0.358084308708253,-1.06395939160588,
9.32883258019174));
#10341=CARTESIAN_POINT('Ctrl Pts',(0.19429771997621,-1.10571128876695,9.35148111779932));
#10342=CARTESIAN_POINT('Ctrl Pts',(0.578041077184206,-0.932257994507511,
9.36869420639422));
#10343=CARTESIAN_POINT('Ctrl Pts',(0.784267005411894,-0.742459747249929,
9.38048462316672));
#10344=CARTESIAN_POINT('Ctrl Pts',(0.912220806450212,-0.586536627035717,
9.38897270741444));
#10345=CARTESIAN_POINT('Ctrl Pts',(1.0759938553963,-0.270623175475007,9.40382440993621));
#10346=CARTESIAN_POINT('Ctrl Pts',(1.09941116997266,0.146857322783328,9.42078900879545));
#10347=CARTESIAN_POINT('Ctrl Pts',(0.953919265860187,0.526219027318657,
9.43775151843459));
#10348=CARTESIAN_POINT('Ctrl Pts',(0.710221272720023,0.851041504230473,
9.45470967792948));
#10349=CARTESIAN_POINT('Ctrl Pts',(0.253020054731783,1.10402529591777,9.47589728129195));
#10350=CARTESIAN_POINT('Ctrl Pts',(-0.372954067823897,1.06874219751822,
9.50131022193773));
#10351=CARTESIAN_POINT('Ctrl Pts',(-0.883802265143228,0.706216247449082,
9.52670835651243));
#10352=CARTESIAN_POINT('Ctrl Pts',(-1.12337158667086,0.127730392023871,
9.55209135669275));
#10353=CARTESIAN_POINT('Ctrl Pts',(-1.01848866350395,-0.489110854542463,
9.57745792779555));
#10354=CARTESIAN_POINT('Ctrl Pts',(-0.60179472455561,-0.955301301450795,
9.60280723074089));
#10355=CARTESIAN_POINT('Ctrl Pts',(-0.001370421070526,-1.12820692400817,
9.62813825936887));
#10356=CARTESIAN_POINT('Ctrl Pts',(0.598555103765798,-0.955298231036643,
9.65345008884992));
#10357=CARTESIAN_POINT('Ctrl Pts',(1.01419982916296,-0.490081317342479,
9.67874178759014));
#10358=CARTESIAN_POINT('Ctrl Pts',(1.11853453908254,0.124451303977719,9.70401243962266));
#10359=CARTESIAN_POINT('Ctrl Pts',(0.880130003500144,0.699796852270577,
9.72926114655504));
#10360=CARTESIAN_POINT('Ctrl Pts',(0.372621603087543,1.05978697679078,9.75448701500854));
#10361=CARTESIAN_POINT('Ctrl Pts',(-0.248041992658389,1.09455009643884,
9.77968916982561));
#10362=CARTESIAN_POINT('Ctrl Pts',(-0.791539658878634,0.79406385342954,
9.80486674471668));
#10363=CARTESIAN_POINT('Ctrl Pts',(-1.0915642463606,0.251016259244287,9.83001890502188));
#10364=CARTESIAN_POINT('Ctrl Pts',(-1.05672913961632,-0.367760770678466,
9.85514476310435));
#10365=CARTESIAN_POINT('Ctrl Pts',(-0.698424490262498,-0.872650684411287,
9.88024361655606));
#10366=CARTESIAN_POINT('Ctrl Pts',(-0.127087637559715,-1.10920064273684,
9.90531437209189));
#10367=CARTESIAN_POINT('Ctrl Pts',(0.481799407328479,-1.00580708103632,
9.93035686134745));
#10368=CARTESIAN_POINT('Ctrl Pts',(0.941725418794725,-0.59448291764376,
9.95536888870454));
#10369=CARTESIAN_POINT('Ctrl Pts',(1.05528916776323,-0.200207605714132,
9.97202614010278));
#10370=CARTESIAN_POINT('Ctrl Pts',(1.05531580562393,-0.00233479057547877,
9.98034674015783));
#10371=CARTESIAN_POINT('Ctrl Pts',(0.932817338094398,0.00223903224158551,
7.22153832457769));
#10372=CARTESIAN_POINT('Ctrl Pts',(0.932793760066264,0.177382610654345,
7.22890315462753));
#10373=CARTESIAN_POINT('Ctrl Pts',(0.832403451678301,0.525794592256776,
7.2436226723496));
#10374=CARTESIAN_POINT('Ctrl Pts',(0.425685989057847,0.889621198330929,
7.26574445281166));
#10375=CARTESIAN_POINT('Ctrl Pts',(-0.112909767544801,0.981053680306889,
7.28789420673005));
#10376=CARTESIAN_POINT('Ctrl Pts',(-0.618460222818951,0.771777784533472,
7.3100782388979));
#10377=CARTESIAN_POINT('Ctrl Pts',(-0.935649120831108,0.324866303046137,
7.33229486959658));
#10378=CARTESIAN_POINT('Ctrl Pts',(-0.966533418354376,-0.223107019260836,
7.35454598288692));
#10379=CARTESIAN_POINT('Ctrl Pts',(-0.700735671162198,-0.704290462461527,
7.37683185460622));
#10380=CARTESIAN_POINT('Ctrl Pts',(-0.218915760021475,-0.970728950195303,
7.39915346188169));
#10381=CARTESIAN_POINT('Ctrl Pts',(0.331698104933367,-0.93994104524836,
7.42151144978389));
#10382=CARTESIAN_POINT('Ctrl Pts',(0.782282737482763,-0.620400150468231,
7.44390658058016));
#10383=CARTESIAN_POINT('Ctrl Pts',(0.994149823047339,-0.109251837914898,
7.46633954009742));
#10384=CARTESIAN_POINT('Ctrl Pts',(0.90145062659539,0.437203917789278,7.48881101627259));
#10385=CARTESIAN_POINT('Ctrl Pts',(0.53155858950099,0.851305491311238,7.51132167468147));
#10386=CARTESIAN_POINT('Ctrl Pts',(-0.00283212755745073,1.00540470537402,
7.53387212978628));
#10387=CARTESIAN_POINT('Ctrl Pts',(-0.538394652874874,0.851310115270327,
7.55646305016228));
#10388=CARTESIAN_POINT('Ctrl Pts',(-0.896468296303925,0.450516088130438,
7.578256674521));
#10389=CARTESIAN_POINT('Ctrl Pts',(-0.998150334469993,-0.0528799063122484,
7.59924871335334));
#10390=CARTESIAN_POINT('Ctrl Pts',(-0.852714766181271,-0.524739769713425,
7.61943418917057));
#10391=CARTESIAN_POINT('Ctrl Pts',(-0.498767893239097,-0.870058344680294,
7.63965341026417));
#10392=CARTESIAN_POINT('Ctrl Pts',(-0.0217992891188254,-1.00474195617444,
7.65990693434088));
#10393=CARTESIAN_POINT('Ctrl Pts',(0.461590577887178,-0.893841791987376,
7.68019475056593));
#10394=CARTESIAN_POINT('Ctrl Pts',(0.897713484577771,-0.511087829973259,
7.70390421214106));
#10395=CARTESIAN_POINT('Ctrl Pts',(1.05284739986986,0.161816435506151,7.73105822118701));
#10396=CARTESIAN_POINT('Ctrl Pts',(0.705905536489394,0.760893081895744,
7.75828300274897));
#10397=CARTESIAN_POINT('Ctrl Pts',(0.172854320016419,1.00020564829781,7.78215786321883));
#10398=CARTESIAN_POINT('Ctrl Pts',(-0.326951940005122,0.96300872535927,
7.8026582555522));
#10399=CARTESIAN_POINT('Ctrl Pts',(-0.713843829504815,0.71294984730384,
7.821483056657));
#10400=CARTESIAN_POINT('Ctrl Pts',(-0.933658986576131,0.362739327222884,
7.83862346287265));
#10401=CARTESIAN_POINT('Ctrl Pts',(-1.00323184902305,-0.0035998581910392,
7.85407042530536));
#10402=CARTESIAN_POINT('Ctrl Pts',(-0.933551814627203,-0.369979955877476,
7.86953812136651));
#10403=CARTESIAN_POINT('Ctrl Pts',(-0.669479465575597,-0.793075720570871,
7.89018956759317));
#10404=CARTESIAN_POINT('Ctrl Pts',(-0.0780371137366919,-1.07927635268795,
7.9160552500025));
#10405=CARTESIAN_POINT('Ctrl Pts',(0.679227399735273,-0.846195851440705,
7.94717855408861));
#10406=CARTESIAN_POINT('Ctrl Pts',(1.0761201749552,-0.158934193380002,7.97838613962336));
#10407=CARTESIAN_POINT('Ctrl Pts',(0.899726434462559,0.617015767811971,
8.00967853755681));
#10408=CARTESIAN_POINT('Ctrl Pts',(0.239950968779785,1.06735347443573,8.04105594349517));
#10409=CARTESIAN_POINT('Ctrl Pts',(-0.462527249163799,0.96075330324454,
8.06902253694048));
#10410=CARTESIAN_POINT('Ctrl Pts',(-0.891570403389457,0.540551941686763,
8.09354880324681));
#10411=CARTESIAN_POINT('Ctrl Pts',(-1.04369474513434,0.0487982002092891,
8.1146091329916));
#10412=CARTESIAN_POINT('Ctrl Pts',(-0.9414272520629,-0.457221001910597,
8.13570732602349));
#10413=CARTESIAN_POINT('Ctrl Pts',(-0.609430038442986,-0.853524812483484,
8.15684347905607));
#10414=CARTESIAN_POINT('Ctrl Pts',(-0.247795399191627,-0.995191046143806,
8.17272380746048));
#10415=CARTESIAN_POINT('Ctrl Pts',(0.00354110646814628,-1.01069610287633,
8.18332260701429));
#10416=CARTESIAN_POINT('Ctrl Pts',(0.171091478472033,-1.00027000944185,
8.19039160004791));
#10417=CARTESIAN_POINT('Ctrl Pts',(0.417066703556737,-0.93784914346088,
8.20100213932378));
#10418=CARTESIAN_POINT('Ctrl Pts',(0.705699028395263,-0.755937475658024,
8.21516517881097));
#10419=CARTESIAN_POINT('Ctrl Pts',(1.01262165785068,-0.343507499055525,
8.2364379486868));
#10420=CARTESIAN_POINT('Ctrl Pts',(1.06497976343805,0.330755715265788,8.26308166354529));
#10421=CARTESIAN_POINT('Ctrl Pts',(0.555379063018134,0.969841090340963,
8.29513806421836));
#10422=CARTESIAN_POINT('Ctrl Pts',(-0.184420846152002,1.08048275305726,
8.32459966541254));
#10423=CARTESIAN_POINT('Ctrl Pts',(-0.764151013947635,0.759084830483624,
8.35144330977293));
#10424=CARTESIAN_POINT('Ctrl Pts',(-1.05294715618884,0.237271017126475,
8.37564898068673));
#10425=CARTESIAN_POINT('Ctrl Pts',(-1.01969845552176,-0.360514646878159,
8.39990064760307));
#10426=CARTESIAN_POINT('Ctrl Pts',(-0.736987911228233,-0.758079682683477,
8.41969861730935));
#10427=CARTESIAN_POINT('Ctrl Pts',(-0.350967168984493,-0.994049689726893,
8.43862194344341));
#10428=CARTESIAN_POINT('Ctrl Pts',(0.0398642534826699,-1.06322766096296,
8.45486200074116));
#10429=CARTESIAN_POINT('Ctrl Pts',(0.461201683510019,-0.949886899588757,
8.47293247966593));
#10430=CARTESIAN_POINT('Ctrl Pts',(0.777368325383777,-0.716895360721043,
8.48921554936968));
#10431=CARTESIAN_POINT('Ctrl Pts',(0.986544217957618,-0.383737196400418,
8.50551849992385));
#10432=CARTESIAN_POINT('Ctrl Pts',(1.07247833681818,0.0677150502151257,
8.52456124674014));
#10433=CARTESIAN_POINT('Ctrl Pts',(0.924204185518489,0.584244428195864,
8.54635705344648));
#10434=CARTESIAN_POINT('Ctrl Pts',(0.472384193043772,0.988084733067928,
8.57092035603831));
#10435=CARTESIAN_POINT('Ctrl Pts',(-0.125803338746724,1.08987257428914,
8.59552639540173));
#10436=CARTESIAN_POINT('Ctrl Pts',(-0.687539065826917,0.857373679191502,
8.62017455944292));
#10437=CARTESIAN_POINT('Ctrl Pts',(-1.04001445832212,0.360821877226519,
8.64486434049305));
#10438=CARTESIAN_POINT('Ctrl Pts',(-1.07436123594458,-0.24816575006392,
8.66959514941773));
#10439=CARTESIAN_POINT('Ctrl Pts',(-0.778947264478789,-0.782953832069739,
8.69436639905966));
#10440=CARTESIAN_POINT('Ctrl Pts',(-0.243432346581132,-1.07907670088945,
8.71917746747984));
#10441=CARTESIAN_POINT('Ctrl Pts',(0.368514215010823,-1.04484341046501,
8.74402771279146));
#10442=CARTESIAN_POINT('Ctrl Pts',(0.869226914069874,-0.68973145530312,
8.76891647464699));
#10443=CARTESIAN_POINT('Ctrl Pts',(1.10461409169443,-0.121791671725091,
8.79384306738233));
#10444=CARTESIAN_POINT('Ctrl Pts',(1.00161987568289,0.485230960329545,8.8188067900524));
#10445=CARTESIAN_POINT('Ctrl Pts',(0.590837878571582,0.945084633471956,
8.84380691007165));
#10446=CARTESIAN_POINT('Ctrl Pts',(-0.00241534456593945,1.11614188043567,
8.86884270930869));
#10447=CARTESIAN_POINT('Ctrl Pts',(-0.596684097120054,0.945119650310722,
8.89391338364207));
#10448=CARTESIAN_POINT('Ctrl Pts',(-0.993843243593392,0.500590727563871,
8.91808845535031));
#10449=CARTESIAN_POINT('Ctrl Pts',(-1.10643245721144,-0.0575015772983971,
8.94136267937612));
#10450=CARTESIAN_POINT('Ctrl Pts',(-0.945619796602633,-0.580262658763286,
8.96373116543371));
#10451=CARTESIAN_POINT('Ctrl Pts',(-0.586107215046292,-0.93104338567574,
8.98425885454782));
#10452=CARTESIAN_POINT('Ctrl Pts',(-0.160798094550997,-1.07909003162016,
9.00293848626054));
#10453=CARTESIAN_POINT('Ctrl Pts',(0.380847821757762,-1.06040707411611,
9.02537151954004));
#10454=CARTESIAN_POINT('Ctrl Pts',(0.85238767414114,-0.740715209958907,
9.04783210789513));
#10455=CARTESIAN_POINT('Ctrl Pts',(1.06757064773678,-0.241674799716118,
9.07031749990356));
#10456=CARTESIAN_POINT('Ctrl Pts',(1.08989480948035,0.30055574321441,9.09281927275907));
#10457=CARTESIAN_POINT('Ctrl Pts',(0.732714846524938,0.921690446594372,
9.12097849776537));
#10458=CARTESIAN_POINT('Ctrl Pts',(0.0475037480025504,1.13202296039076,
9.14917647651982));
#10459=CARTESIAN_POINT('Ctrl Pts',(-0.47863811734372,0.989412084764905,
9.17175595217751));
#10460=CARTESIAN_POINT('Ctrl Pts',(-0.844340163433761,0.720354496408093,
9.19058402886265));
#10461=CARTESIAN_POINT('Ctrl Pts',(-1.08711624461903,0.275017683314028,
9.21131102491027));
#10462=CARTESIAN_POINT('Ctrl Pts',(-1.08678177842939,-0.278315106506191,
9.23393881798215));
#10463=CARTESIAN_POINT('Ctrl Pts',(-0.822280508726689,-0.765009547413839,
9.25658444333911));
#10464=CARTESIAN_POINT('Ctrl Pts',(-0.356463083692494,-1.06542928247866,
9.27924670945844));
#10465=CARTESIAN_POINT('Ctrl Pts',(0.196587215171616,-1.10729173992762,
9.30192398401361));
#10466=CARTESIAN_POINT('Ctrl Pts',(0.581247622139915,-0.933498715306414,
9.31918146203166));
#10467=CARTESIAN_POINT('Ctrl Pts',(0.78805035283314,-0.743174183407583,
9.33100500669254));
#10468=CARTESIAN_POINT('Ctrl Pts',(0.916397144732695,-0.586774635437394,
9.339519544202));
#10469=CARTESIAN_POINT('Ctrl Pts',(1.08075456481652,-0.269770476008509,
9.35442396179574));
#10470=CARTESIAN_POINT('Ctrl Pts',(1.1043406223813,0.149554271447882,9.37146787576897));
#10471=CARTESIAN_POINT('Ctrl Pts',(0.958119700633825,0.530862407294559,
9.38851799488734));
#10472=CARTESIAN_POINT('Ctrl Pts',(0.713059280154455,0.857531088386705,
9.4055734547437));
#10473=CARTESIAN_POINT('Ctrl Pts',(0.252911145537254,1.11223884436659,9.42690335124296));
#10474=CARTESIAN_POINT('Ctrl Pts',(-0.377817110739569,1.07678655749214,
9.45251244753617));
#10475=CARTESIAN_POINT('Ctrl Pts',(-0.893151735400408,0.711201885990653,
9.47813454118543));
#10476=CARTESIAN_POINT('Ctrl Pts',(-1.13514464160495,0.12712014183053,9.50376820319782));
#10477=CARTESIAN_POINT('Ctrl Pts',(-1.0292241515188,-0.496405026542247,
9.52941250474413));
#10478=CARTESIAN_POINT('Ctrl Pts',(-0.607651992297783,-0.968196730147786,
9.55506626992792));
#10479=CARTESIAN_POINT('Ctrl Pts',(0.000516788824355856,-1.14343121492963,
9.58072843587768));
#10480=CARTESIAN_POINT('Ctrl Pts',(0.608868148912967,-0.968192123375259,
9.60639786060031));
#10481=CARTESIAN_POINT('Ctrl Pts',(1.03084013393238,-0.496034157006386,
9.63207344185143));
#10482=CARTESIAN_POINT('Ctrl Pts',(1.13694700570821,0.128377444332003,9.6577540442593));
#10483=CARTESIAN_POINT('Ctrl Pts',(0.894542209160189,0.713620555570391,
9.68343855267843));
#10484=CARTESIAN_POINT('Ctrl Pts',(0.377864659011472,1.08022831008716,9.70912582606619));
#10485=CARTESIAN_POINT('Ctrl Pts',(-0.254708500473694,1.11575062973695,
9.73481475003169));
#10486=CARTESIAN_POINT('Ctrl Pts',(-0.809235469376882,0.809269589714066,
9.76050416245622));
#10487=CARTESIAN_POINT('Ctrl Pts',(-1.11570364867539,0.254741293244564,
9.78619302028867));
#10488=CARTESIAN_POINT('Ctrl Pts',(-1.08017949873475,-0.377791903239077,
9.81187998879018));
#10489=CARTESIAN_POINT('Ctrl Pts',(-0.71362254477927,-0.894447905725997,
9.83756442934909));
#10490=CARTESIAN_POINT('Ctrl Pts',(-0.12848878406753,-1.13680446508768,
9.86324414525839));
#10491=CARTESIAN_POINT('Ctrl Pts',(0.495751120741053,-1.03087493259538,
9.88892046721288));
#10492=CARTESIAN_POINT('Ctrl Pts',(0.967762675373715,-0.608896178670159,
9.91458687730015));
#10493=CARTESIAN_POINT('Ctrl Pts',(1.08449349913632,-0.20388861139028,9.93170092751877));
#10494=CARTESIAN_POINT('Ctrl Pts',(1.08452085900721,-0.000652520652106218,
9.94024705461864));
#10495=CARTESIAN_POINT('Ctrl Pts',(0.916384184646393,-0.000812414047608488,
7.294052389051));
#10496=CARTESIAN_POINT('Ctrl Pts',(0.91636102789669,0.171201801238968,7.30128562862064));
#10497=CARTESIAN_POINT('Ctrl Pts',(0.817714321229081,0.513121139438122,
7.31573445825018));
#10498=CARTESIAN_POINT('Ctrl Pts',(0.419183940001587,0.869421294661586,
7.33740687562125));
#10499=CARTESIAN_POINT('Ctrl Pts',(-0.107511678749076,0.958699494084228,
7.35906851046912));
#10500=CARTESIAN_POINT('Ctrl Pts',(-0.600919896114351,0.754308982034972,
7.38072396635307));
#10501=CARTESIAN_POINT('Ctrl Pts',(-0.90986434389333,0.318796907723617,
7.40237277329793));
#10502=CARTESIAN_POINT('Ctrl Pts',(-0.939775508284088,-0.214171715938281,
7.42401675026896));
#10503=CARTESIAN_POINT('Ctrl Pts',(-0.681599841371247,-0.681292688788261,
7.44565670173072));
#10504=CARTESIAN_POINT('Ctrl Pts',(-0.214544410932947,-0.939420652432807,
7.46729389336328));
#10505=CARTESIAN_POINT('Ctrl Pts',(0.318210121393327,-0.909504154003217,
7.48892939490667));
#10506=CARTESIAN_POINT('Ctrl Pts',(0.753380323755671,-0.600740800554072,
7.51056436224741));
#10507=CARTESIAN_POINT('Ctrl Pts',(0.957580132215121,-0.107767532236841,
7.53219991215366));
#10508=CARTESIAN_POINT('Ctrl Pts',(0.868211541183081,0.418326077149899,
7.55383719616653));
#10509=CARTESIAN_POINT('Ctrl Pts',(0.512571933875558,0.816291655068875,
7.5754773236975));
#10510=CARTESIAN_POINT('Ctrl Pts',(-0.000319842256805562,0.964068440570839,
7.59712147475655));
#10511=CARTESIAN_POINT('Ctrl Pts',(-0.513473050755741,0.816299802289933,
7.61877069085977));
#10512=CARTESIAN_POINT('Ctrl Pts',(-0.855981669773446,0.432764156671664,
7.63962426478969));
#10513=CARTESIAN_POINT('Ctrl Pts',(-0.953048966078777,-0.0481973160739187,
7.65968184621655));
#10514=CARTESIAN_POINT('Ctrl Pts',(-0.814207366238296,-0.498404503042273,
7.67894394873332));
#10515=CARTESIAN_POINT('Ctrl Pts',(-0.476868785727358,-0.827423916195667,
7.69821324881017));
#10516=CARTESIAN_POINT('Ctrl Pts',(-0.0229026114670843,-0.955530455908849,
7.71749025791405));
#10517=CARTESIAN_POINT('Ctrl Pts',(0.436569596441587,-0.85005354508792,
7.73677624340631));
#10518=CARTESIAN_POINT('Ctrl Pts',(0.850579801372237,-0.486583791265893,
7.75928808298809));
#10519=CARTESIAN_POINT('Ctrl Pts',(0.997455702178448,0.151411719541167,
7.7850346645544));
#10520=CARTESIAN_POINT('Ctrl Pts',(0.66892061877028,0.718298327157484,7.81080466018562));
#10521=CARTESIAN_POINT('Ctrl Pts',(0.165105277263114,0.944401326593409,
7.83337036699914));
#10522=CARTESIAN_POINT('Ctrl Pts',(-0.306760321133552,0.909226016129731,
7.85272560376473));
#10523=CARTESIAN_POINT('Ctrl Pts',(-0.671629161971406,0.673332022752352,
7.87048190618396));
#10524=CARTESIAN_POINT('Ctrl Pts',(-0.878741185245582,0.343312833427155,
7.88663430695027));
#10525=CARTESIAN_POINT('Ctrl Pts',(-0.94423011831239,-0.00164456370475496,
7.90118025371029));
#10526=CARTESIAN_POINT('Ctrl Pts',(-0.878646080781751,-0.346381218378189,
7.91573520582742));
#10527=CARTESIAN_POINT('Ctrl Pts',(-0.630315057219919,-0.74419509882429,
7.93515396976183));
#10528=CARTESIAN_POINT('Ctrl Pts',(-0.0746840041171197,-1.01290792724034,
7.95945317547552));
#10529=CARTESIAN_POINT('Ctrl Pts',(0.635655594458093,-0.79408428312529,
7.98865203565831));
#10530=CARTESIAN_POINT('Ctrl Pts',(1.00738408651088,-0.150077117453577,
8.01789434930099));
#10531=CARTESIAN_POINT('Ctrl Pts',(0.842150637204844,0.576077696538741,
8.04718205840345));
#10532=CARTESIAN_POINT('Ctrl Pts',(0.225271464949242,0.996955646093593,
8.07651744286865));
#10533=CARTESIAN_POINT('Ctrl Pts',(-0.43077106632299,0.897282204130466,
8.10263821657078));
#10534=CARTESIAN_POINT('Ctrl Pts',(-0.831114549612531,0.505125213112986,
8.12552681825321));
#10535=CARTESIAN_POINT('Ctrl Pts',(-0.972961487683506,0.0464809015971219,
8.14516966456063));
#10536=CARTESIAN_POINT('Ctrl Pts',(-0.877602512982472,-0.425191958105245,
8.16483693107729));
#10537=CARTESIAN_POINT('Ctrl Pts',(-0.568276019795686,-0.794384958085934,
8.18452868985693));
#10538=CARTESIAN_POINT('Ctrl Pts',(-0.231513901591766,-0.926289452386036,
8.19931732873309));
#10539=CARTESIAN_POINT('Ctrl Pts',(0.00245799136279632,-0.940722053136144,
8.20918392331538));
#10540=CARTESIAN_POINT('Ctrl Pts',(0.158416318109175,-0.931017174660892,
8.21576392644465));
#10541=CARTESIAN_POINT('Ctrl Pts',(0.387337229899669,-0.872920481534924,
8.22563902104255));
#10542=CARTESIAN_POINT('Ctrl Pts',(0.655887282970169,-0.703657924089153,
8.23881727887628));
#10543=CARTESIAN_POINT('Ctrl Pts',(0.941363930700124,-0.320023744551051,
8.25860467543646));
#10544=CARTESIAN_POINT('Ctrl Pts',(0.98998838540909,0.306890866588042,8.28337764757458));
#10545=CARTESIAN_POINT('Ctrl Pts',(0.516353784183733,0.900777750505931,
8.31317026550616));
#10546=CARTESIAN_POINT('Ctrl Pts',(-0.170895376698677,1.00351776465295,
8.34053992286506));
#10547=CARTESIAN_POINT('Ctrl Pts',(-0.709276893706946,0.705023452750632,
8.36547008485353));
#10548=CARTESIAN_POINT('Ctrl Pts',(-0.977416665651329,0.220507453202623,
8.38794586803964));
#10549=CARTESIAN_POINT('Ctrl Pts',(-0.946540072103369,-0.334455386118879,
8.41046071721602));
#10550=CARTESIAN_POINT('Ctrl Pts',(-0.68410690604905,-0.703498657680165,
8.42883889692179));
#10551=CARTESIAN_POINT('Ctrl Pts',(-0.325798798725742,-0.922527998573711,
8.44640383700852));
#10552=CARTESIAN_POINT('Ctrl Pts',(0.0369623652280897,-0.986736749875426,
8.46147757987718));
#10553=CARTESIAN_POINT('Ctrl Pts',(0.428035342802407,-0.881538480517849,
8.47825020517938));
#10554=CARTESIAN_POINT('Ctrl Pts',(0.721493797857177,-0.665282361395511,
8.49336377211604));
#10555=CARTESIAN_POINT('Ctrl Pts',(0.915653860248132,-0.356045284728461,
8.50849631732876));
#10556=CARTESIAN_POINT('Ctrl Pts',(0.995424601695212,0.0630116385503096,
8.52617266101546));
#10557=CARTESIAN_POINT('Ctrl Pts',(0.857789064698206,0.542518419007572,
8.54640619473492));
#10558=CARTESIAN_POINT('Ctrl Pts',(0.438308728778306,0.917473083752972,
8.56921188084219));
#10559=CARTESIAN_POINT('Ctrl Pts',(-0.117171435160921,1.01201202635041,
8.59206127082509));
#10560=CARTESIAN_POINT('Ctrl Pts',(-0.638927134962905,0.79608335109431,
8.61495471428855));
#10561=CARTESIAN_POINT('Ctrl Pts',(-0.966415516773689,0.334773910945176,
8.63789269515097));
#10562=CARTESIAN_POINT('Ctrl Pts',(-0.99836233251678,-0.231176077678445,
8.66087559759738));
#10563=CARTESIAN_POINT('Ctrl Pts',(-0.723758542776752,-0.72835451264945,
8.68390381202748));
#10564=CARTESIAN_POINT('Ctrl Pts',(-0.2257474509395,-1.00377738419217,8.70697768864429));
#10565=CARTESIAN_POINT('Ctrl Pts',(0.343600136828314,-0.971963977022025,
8.73009755919227));
#10566=CARTESIAN_POINT('Ctrl Pts',(0.809690300867129,-0.641455706076566,
8.75326372412054));
#10567=CARTESIAN_POINT('Ctrl Pts',(1.02893814149207,-0.112569327400558,
8.77647646087813));
#10568=CARTESIAN_POINT('Ctrl Pts',(0.933018095440899,0.453037359706394,
8.79973601914518));
#10569=CARTESIAN_POINT('Ctrl Pts',(0.550088474279159,0.881786204706492,
8.82304262430822));
#10570=CARTESIAN_POINT('Ctrl Pts',(-0.00331223803182207,1.04140779084441,
8.84639646939416));
#10571=CARTESIAN_POINT('Ctrl Pts',(-0.558044053109453,0.881822628119523,
8.86979773274531));
#10572=CARTESIAN_POINT('Ctrl Pts',(-0.929061567856926,0.46663875567079,
8.89237806561174));
#10573=CARTESIAN_POINT('Ctrl Pts',(-1.03434228395829,-0.0550007789708017,
8.91413164432233));
#10574=CARTESIAN_POINT('Ctrl Pts',(-0.883973293660551,-0.543961856211894,
8.93505289544298));
#10575=CARTESIAN_POINT('Ctrl Pts',(-0.547515238324857,-0.872307713095914,
8.95426532130326));
#10576=CARTESIAN_POINT('Ctrl Pts',(-0.149203363966445,-1.01097948256328,
8.97175868300262));
#10577=CARTESIAN_POINT('Ctrl Pts',(0.358343864201227,-0.993501252395768,
8.99277925477119));
#10578=CARTESIAN_POINT('Ctrl Pts',(0.800624893951803,-0.693778031940356,
9.01384209964755));
#10579=CARTESIAN_POINT('Ctrl Pts',(1.00264542737942,-0.225346188642404,
9.03494770829309));
#10580=CARTESIAN_POINT('Ctrl Pts',(1.02364288737243,0.283933103839578,9.05608172922299));
#10581=CARTESIAN_POINT('Ctrl Pts',(0.688000806473435,0.867935649292769,
9.08255185043447));
#10582=CARTESIAN_POINT('Ctrl Pts',(0.0430534476606014,1.06608732574115,
9.10909256714991));
#10583=CARTESIAN_POINT('Ctrl Pts',(-0.452738363714565,0.93174161838465,
9.13036778259929));
#10584=CARTESIAN_POINT('Ctrl Pts',(-0.797580117742964,0.678064020635429,
9.14812059831063));
#10585=CARTESIAN_POINT('Ctrl Pts',(-1.02673710165334,0.257847579606903,
9.16767814991022));
#10586=CARTESIAN_POINT('Ctrl Pts',(-1.02648106844828,-0.264826941713865,
9.18905154450334));
#10587=CARTESIAN_POINT('Ctrl Pts',(-0.776460073134754,-0.725026353915674,
9.21046173226614));
#10588=CARTESIAN_POINT('Ctrl Pts',(-0.33562848698493,-1.00940897138283,
9.23190879544451));
#10589=CARTESIAN_POINT('Ctrl Pts',(0.188329899581691,-1.0491402456296,9.25339297598941));
#10590=CARTESIAN_POINT('Ctrl Pts',(0.553136534120908,-0.884368968829443,
9.26975676409425));
#10591=CARTESIAN_POINT('Ctrl Pts',(0.749404683996913,-0.703743773738387,
9.28097769251118));
#10592=CARTESIAN_POINT('Ctrl Pts',(0.871248898640151,-0.555270911284687,
9.28906053551857));
#10593=CARTESIAN_POINT('Ctrl Pts',(1.02735904501533,-0.254207860668812,
9.30321546934299));
#10594=CARTESIAN_POINT('Ctrl Pts',(1.04984503084766,0.144376165230818,9.31941439398456));
#10595=CARTESIAN_POINT('Ctrl Pts',(0.910732980180467,0.507198490051187,
9.33563696536372));
#10596=CARTESIAN_POINT('Ctrl Pts',(0.677430691215826,0.818220810897905,
9.3518744741977));
#10597=CARTESIAN_POINT('Ctrl Pts',(0.238978705298457,1.0610211403517,9.37219870850224));
#10598=CARTESIAN_POINT('Ctrl Pts',(-0.362859301163257,1.02730471082093,
9.39663266712745));
#10599=CARTESIAN_POINT('Ctrl Pts',(-0.855287575123984,0.678104309011124,
9.42111055993154));
#10600=CARTESIAN_POINT('Ctrl Pts',(-1.08690633568849,0.119360359866055,
9.44563212936705));
#10601=CARTESIAN_POINT('Ctrl Pts',(-0.98555083882038,-0.47798510234353,
9.47019679120956));
#10602=CARTESIAN_POINT('Ctrl Pts',(-0.581229979579629,-0.930648430527953,
9.49480407397801));
#10603=CARTESIAN_POINT('Ctrl Pts',(0.00295283093870749,-1.09909733418053,
9.51945343242555));
#10604=CARTESIAN_POINT('Ctrl Pts',(0.588197155365154,-0.930641683598714,
9.54414431358483));
#10605=CARTESIAN_POINT('Ctrl Pts',(0.994786308140254,-0.475881984543007,
9.56887614236257));
#10606=CARTESIAN_POINT('Ctrl Pts',(1.09727215135844,0.126473271551238,9.59364831685043));
#10607=CARTESIAN_POINT('Ctrl Pts',(0.863198931394216,0.691932043003254,
9.61846022152596));
#10608=CARTESIAN_POINT('Ctrl Pts',(0.363371458512755,1.04674092501543,9.64331120732547));
#10609=CARTESIAN_POINT('Ctrl Pts',(-0.249563746611437,1.08129056426141,
9.66820062239446));
#10610=CARTESIAN_POINT('Ctrl Pts',(-0.787750701358366,0.78399163290601,
9.69312775992718));
#10611=CARTESIAN_POINT('Ctrl Pts',(-1.0857205254415,0.245119969922457,9.71809198124987));
#10612=CARTESIAN_POINT('Ctrl Pts',(-1.05128010206474,-0.370570820675122,
9.74309241562914));
#10613=CARTESIAN_POINT('Ctrl Pts',(-0.694056959651085,-0.874314390372112,
9.76812867801744));
#10614=CARTESIAN_POINT('Ctrl Pts',(-0.122812930922393,-1.11106608042246,
9.79319923890406));
#10615=CARTESIAN_POINT('Ctrl Pts',(0.487625669319352,-1.007614700358,9.81830510245824));
#10616=CARTESIAN_POINT('Ctrl Pts',(0.950000744760197,-0.594415484013305,
9.84344158104869));
#10617=CARTESIAN_POINT('Ctrl Pts',(1.06455322262812,-0.197156271448973,
9.86022677005009));
#10618=CARTESIAN_POINT('Ctrl Pts',(1.06458008203471,0.00236224302569044,
9.86861657216291));
#10619=CARTESIAN_POINT('Ctrl Pts',(0.962718230280815,-0.00325963339072736,
7.35239823212382));
#10620=CARTESIAN_POINT('Ctrl Pts',(0.96269391832364,0.177335756254699,7.35999231216134));
#10621=CARTESIAN_POINT('Ctrl Pts',(0.859091395002888,0.536367440659574,
7.37516300480678));
#10622=CARTESIAN_POINT('Ctrl Pts',(0.441244001169262,0.909763722620838,
7.39787937610872));
#10623=CARTESIAN_POINT('Ctrl Pts',(-0.110083694811868,1.0031262480341,7.42055272981597));
#10624=CARTESIAN_POINT('Ctrl Pts',(-0.625739413289849,0.789385321248754,
7.44318475760545));
#10625=CARTESIAN_POINT('Ctrl Pts',(-0.94804788351903,0.334822437451381,
7.46577552364345));
#10626=CARTESIAN_POINT('Ctrl Pts',(-0.979088619717144,-0.220522420853946,
7.48832585783457));
#10627=CARTESIAN_POINT('Ctrl Pts',(-0.710391608174497,-0.706415596651747,
7.51083627889516));
#10628=CARTESIAN_POINT('Ctrl Pts',(-0.225225071456474,-0.97440720732087,
7.53330747523763));
#10629=CARTESIAN_POINT('Ctrl Pts',(0.327204367923681,-0.943256814728376,
7.55574009450392));
#10630=CARTESIAN_POINT('Ctrl Pts',(0.777625996912355,-0.623512949022436,
7.57813482755551));
#10631=CARTESIAN_POINT('Ctrl Pts',(0.988540004465044,-0.113987597368397,
7.60049237934514));
#10632=CARTESIAN_POINT('Ctrl Pts',(0.896206941446668,0.4287655787072,7.62281347470688));
#10633=CARTESIAN_POINT('Ctrl Pts',(0.529825699099087,0.838550426236005,
7.64509886891068));
#10634=CARTESIAN_POINT('Ctrl Pts',(0.00247375335561738,0.990354343679899,
7.66734929755787));
#10635=CARTESIAN_POINT('Ctrl Pts',(-0.524138115921198,0.838567973237236,
7.68956560662869));
#10636=CARTESIAN_POINT('Ctrl Pts',(-0.874927095876008,0.44556549648226,
7.71092685158314));
#10637=CARTESIAN_POINT('Ctrl Pts',(-0.974100408150317,-0.0463432791829163,
7.73143835597165));
#10638=CARTESIAN_POINT('Ctrl Pts',(-0.832242715660948,-0.506006054432365,
7.75110411184544));
#10639=CARTESIAN_POINT('Ctrl Pts',(-0.488286707768319,-0.841336359336464,
7.77074553879654));
#10640=CARTESIAN_POINT('Ctrl Pts',(-0.0262305298762631,-0.971625611540388,
7.79036342458605));
#10641=CARTESIAN_POINT('Ctrl Pts',(0.440601778900192,-0.864355709837979,
7.80995806390901));
#10642=CARTESIAN_POINT('Ctrl Pts',(0.860506937013534,-0.495559957146942,
7.83279185554976));
#10643=CARTESIAN_POINT('Ctrl Pts',(1.00887636243662,0.150329159697506,7.8588498166984));
#10644=CARTESIAN_POINT('Ctrl Pts',(0.676895321423857,0.722550287249622,
7.88486552355294));
#10645=CARTESIAN_POINT('Ctrl Pts',(0.169196097474721,0.950263594233254,
7.90760172054666));
#10646=CARTESIAN_POINT('Ctrl Pts',(-0.305463577404435,0.914780507645835,
7.9270708861676));
#10647=CARTESIAN_POINT('Ctrl Pts',(-0.671810169761784,0.677822910309403,
7.94489953704969));
#10648=CARTESIAN_POINT('Ctrl Pts',(-0.879447912476032,0.346878272400615,
7.96109498578419));
#10649=CARTESIAN_POINT('Ctrl Pts',(-0.944987627577209,0.00140801812198339,
7.97566103547143));
#10650=CARTESIAN_POINT('Ctrl Pts',(-0.879352813477502,-0.343383692137119,
7.99021763892266));
#10651=CARTESIAN_POINT('Ctrl Pts',(-0.631225667469588,-0.740751352130975,
8.00961452012653));
#10652=CARTESIAN_POINT('Ctrl Pts',(-0.0771397493560771,-1.00839347936742,
8.03383644726459));
#10653=CARTESIAN_POINT('Ctrl Pts',(0.629177191130674,-0.790429234820235,
8.06287098714952));
#10654=CARTESIAN_POINT('Ctrl Pts',(0.997610200365256,-0.151417910261682,
8.09187470557712));
#10655=CARTESIAN_POINT('Ctrl Pts',(0.833777198875691,0.56702235109786,8.12085049620515));
#10656=CARTESIAN_POINT('Ctrl Pts',(0.224721714435626,0.982134093303416,
8.14980096634948));
#10657=CARTESIAN_POINT('Ctrl Pts',(-0.421115897262969,0.883719661262009,
8.17551361664085));
#10658=CARTESIAN_POINT('Ctrl Pts',(-0.814372361173212,0.498341989081361,
8.19800033305438));
#10659=CARTESIAN_POINT('Ctrl Pts',(-0.953427319669304,0.0484314344791073,
8.21726600639097));
#10660=CARTESIAN_POINT('Ctrl Pts',(-0.859948384303787,-0.413455741489949,
8.23652418724655));
#10661=CARTESIAN_POINT('Ctrl Pts',(-0.557437339114465,-0.774372047655641,
8.25577651913894));
#10662=CARTESIAN_POINT('Ctrl Pts',(-0.228690647482073,-0.903055243520952,
8.27021029594821));
#10663=CARTESIAN_POINT('Ctrl Pts',(-0.000515736396863631,-0.917128271832189,
8.27983239822654));
#10664=CARTESIAN_POINT('Ctrl Pts',(0.151517914219297,-0.907666032608045,
8.28624658587932));
#10665=CARTESIAN_POINT('Ctrl Pts',(0.374537923474286,-0.851052981986712,
8.29586674787202));
#10666=CARTESIAN_POINT('Ctrl Pts',(0.635885574200474,-0.686297071615076,
8.30869123230048));
#10667=CARTESIAN_POINT('Ctrl Pts',(0.913362706304005,-0.31330570504482,
8.32792585459235));
#10668=CARTESIAN_POINT('Ctrl Pts',(0.960298111398029,0.295105768078741,
8.35196483325124));
#10669=CARTESIAN_POINT('Ctrl Pts',(0.501465375120066,0.869873888531251,
8.38080476513217));
#10670=CARTESIAN_POINT('Ctrl Pts',(-0.162449147078619,0.968850911622415,
8.40724050705978));
#10671=CARTESIAN_POINT('Ctrl Pts',(-0.681456260321231,0.680932154126198,
8.43127468009259));
#10672=CARTESIAN_POINT('Ctrl Pts',(-0.939460097390127,0.214496687258891,
8.45290679063804));
#10673=CARTESIAN_POINT('Ctrl Pts',(-0.909663908454563,-0.318827476974102,
8.47454207053821));
#10674=CARTESIAN_POINT('Ctrl Pts',(-0.657794745513012,-0.672857183575831,
8.49217320723589));
#10675=CARTESIAN_POINT('Ctrl Pts',(-0.314367073536956,-0.882767599732077,
8.50900742283414));
#10676=CARTESIAN_POINT('Ctrl Pts',(0.0329724123550007,-0.944188244476581,
8.52343929983286));
#10677=CARTESIAN_POINT('Ctrl Pts',(0.406941645978025,-0.843550008334516,
8.53947768998332));
#10678=CARTESIAN_POINT('Ctrl Pts',(0.687288910638273,-0.636918632610979,
8.55391643183634));
#10679=CARTESIAN_POINT('Ctrl Pts',(0.872566467708324,-0.341764473236915,
8.56835770756406));
#10680=CARTESIAN_POINT('Ctrl Pts',(0.948591468806281,0.0578163985634961,
8.58521127785539));
#10681=CARTESIAN_POINT('Ctrl Pts',(0.817421234004075,0.514441347046019,
8.60447819513267));
#10682=CARTESIAN_POINT('Ctrl Pts',(0.418417535373532,0.870947360259675,
8.62616498275342));
#10683=CARTESIAN_POINT('Ctrl Pts',(-0.109148101016243,0.960627692910106,
8.64786339052937));
#10684=CARTESIAN_POINT('Ctrl Pts',(-0.603968507622487,0.755735717138706,
8.66957489683606));
#10685=CARTESIAN_POINT('Ctrl Pts',(-0.914090995977477,0.318717601643026,
8.69130039086325));
#10686=CARTESIAN_POINT('Ctrl Pts',(-0.944218013863038,-0.216688417589151,
8.7130410220435));
#10687=CARTESIAN_POINT('Ctrl Pts',(-0.68467496995104,-0.686407268559419,
8.73479781719363));
#10688=CARTESIAN_POINT('Ctrl Pts',(-0.214641641910551,-0.946254378190861,
8.75657184998439));
#10689=CARTESIAN_POINT('Ctrl Pts',(0.322046159483052,-0.916178478730096,
8.77836416626867));
#10690=CARTESIAN_POINT('Ctrl Pts',(0.760864759580575,-0.60490496580893,
8.80017580379087));
#10691=CARTESIAN_POINT('Ctrl Pts',(0.967009403930397,-0.107413789658448,
8.8220077929034));
#10692=CARTESIAN_POINT('Ctrl Pts',(0.876805004086599,0.424019495378302,
8.84386114484036));
#10693=CARTESIAN_POINT('Ctrl Pts',(0.517305794945177,0.826421245036036,
8.86573687513684));
#10694=CARTESIAN_POINT('Ctrl Pts',(-0.00167454613960216,0.9760401976625,
8.8876359334133));
#10695=CARTESIAN_POINT('Ctrl Pts',(-0.521385932264157,0.826457735334773,
8.9095593580425));
#10696=CARTESIAN_POINT('Ctrl Pts',(-0.868640455956031,0.43777148600058,
8.93069501819422));
#10697=CARTESIAN_POINT('Ctrl Pts',(-0.967067305884696,-0.0501482616685878,
8.95104098324805));
#10698=CARTESIAN_POINT('Ctrl Pts',(-0.82647974711531,-0.507164794805139,
8.97059532406617));
#10699=CARTESIAN_POINT('Ctrl Pts',(-0.5121841740472,-0.813829042722063,
8.98854003426641));
#10700=CARTESIAN_POINT('Ctrl Pts',(-0.140348873654308,-0.943265643944857,
9.00486969124519));
#10701=CARTESIAN_POINT('Ctrl Pts',(0.333244783959833,-0.926930320777186,
9.02448345024546));
#10702=CARTESIAN_POINT('Ctrl Pts',(0.7456134311321,-0.6473862729714,9.04412252713801));
#10703=CARTESIAN_POINT('Ctrl Pts',(0.933852231346841,-0.210851073850686,
9.06379015343548));
#10704=CARTESIAN_POINT('Ctrl Pts',(0.953394997791234,0.263570308883686,
9.08347689733712));
#10705=CARTESIAN_POINT('Ctrl Pts',(0.640831730089639,0.807240118677375,
9.10811933138053));
#10706=CARTESIAN_POINT('Ctrl Pts',(0.0407574010195053,0.991527955790331,
9.13281136872211));
#10707=CARTESIAN_POINT('Ctrl Pts',(-0.420321639507707,0.866574252716919,
9.15259677633439));
#10708=CARTESIAN_POINT('Ctrl Pts',(-0.740930835144724,0.630710272872244,
9.16910201499638));
#10709=CARTESIAN_POINT('Ctrl Pts',(-0.953906223882338,0.240129411046737,
9.18727911280356));
#10710=CARTESIAN_POINT('Ctrl Pts',(-0.953649235823561,-0.245530083594935,
9.20713863170929));
#10711=CARTESIAN_POINT('Ctrl Pts',(-0.721385076575375,-0.673014021182606,
9.22702670918586));
#10712=CARTESIAN_POINT('Ctrl Pts',(-0.311975189904776,-0.937107659022901,
9.24694424499692));
#10713=CARTESIAN_POINT('Ctrl Pts',(0.174531516569616,-0.973987841354782,
9.26689261090667));
#10714=CARTESIAN_POINT('Ctrl Pts',(0.513193794898759,-0.821012780675783,
9.2820833145985));
#10715=CARTESIAN_POINT('Ctrl Pts',(0.695385853961652,-0.653341121506572,
9.29249948482213));
#10716=CARTESIAN_POINT('Ctrl Pts',(0.808487412662864,-0.515520951601559,
9.3000023335951));
#10717=CARTESIAN_POINT('Ctrl Pts',(0.953387192260482,-0.236072454603558,
9.31314087645884));
#10718=CARTESIAN_POINT('Ctrl Pts',(0.974249964060649,0.133859198164401,
9.32817495318504));
#10719=CARTESIAN_POINT('Ctrl Pts',(0.845142220453277,0.470585978846416,
9.34323069547589));
#10720=CARTESIAN_POINT('Ctrl Pts',(0.628623531777474,0.759231089356386,
9.35829990911351));
#10721=CARTESIAN_POINT('Ctrl Pts',(0.221724378384738,0.984555659606961,
9.37716126766761));
#10722=CARTESIAN_POINT('Ctrl Pts',(-0.336811565884306,0.953266271395749,
9.39983708161437));
#10723=CARTESIAN_POINT('Ctrl Pts',(-0.793838921575871,0.629175078952241,
9.42255501604705));
#10724=CARTESIAN_POINT('Ctrl Pts',(-1.00883395642591,0.110553388403418,
9.44531583505166));
#10725=CARTESIAN_POINT('Ctrl Pts',(-0.914753666531486,-0.443981321671508,
9.4681199191005));
#10726=CARTESIAN_POINT('Ctrl Pts',(-0.53935346555354,-0.864287702720483,
9.49096779294908));
#10727=CARTESIAN_POINT('Ctrl Pts',(0.00317473919602999,-1.02074393938534,
9.51385987936846));
#10728=CARTESIAN_POINT('Ctrl Pts',(0.546842451951703,-0.864277453369769,
9.53679662034949));
#10729=CARTESIAN_POINT('Ctrl Pts',(0.924675422089117,-0.441717222447211,
9.55977841069135));
#10730=CARTESIAN_POINT('Ctrl Pts',(1.01996808440899,0.118196481355525,9.58280563347303));
#10731=CARTESIAN_POINT('Ctrl Pts',(0.802331121841736,0.64402993935177,9.6058786398591));
#10732=CARTESIAN_POINT('Ctrl Pts',(0.337364397173406,0.974133999160165,
9.62899775887225));
#10733=CARTESIAN_POINT('Ctrl Pts',(-0.233104637031958,1.00632652768241,
9.65216329850443));
#10734=CARTESIAN_POINT('Ctrl Pts',(-0.734273786426299,0.729521681583079,
9.67537552627366));
#10735=CARTESIAN_POINT('Ctrl Pts',(-1.01192271602118,0.227485149733832,
9.69863471831026));
#10736=CARTESIAN_POINT('Ctrl Pts',(-0.979861010625463,-0.346471505307732,
9.72194105790298));
#10737=CARTESIAN_POINT('Ctrl Pts',(-0.646687232733913,-0.816385458535924,
9.74529485019366));
#10738=CARTESIAN_POINT('Ctrl Pts',(-0.113515831859443,-1.03740747700115,
9.76869605816828));
#10739=CARTESIAN_POINT('Ctrl Pts',(0.45666043399166,-0.940854540198569,
9.79214533421283));
#10740=CARTESIAN_POINT('Ctrl Pts',(0.888877742368337,-0.554658268165104,
9.8156417140768));
#10741=CARTESIAN_POINT('Ctrl Pts',(0.996072925475586,-0.183171021132321,
9.83133914183944));
#10742=CARTESIAN_POINT('Ctrl Pts',(0.996098069974061,0.00360871894456211,
9.83919327538718));
#10743=CARTESIAN_POINT('Ctrl Pts',(1.03719675406882,-0.00324058202589225,
7.35218360836862));
#10744=CARTESIAN_POINT('Ctrl Pts',(1.03717058144385,0.191176320370734,7.36035888637736));
#10745=CARTESIAN_POINT('Ctrl Pts',(0.925557853409022,0.578088834603603,
7.37670781473685));
#10746=CARTESIAN_POINT('Ctrl Pts',(0.47537110567802,0.980347295995417,7.40118088192312));
#10747=CARTESIAN_POINT('Ctrl Pts',(-0.118659904383316,1.08096987560822,
7.42561186891184));
#10748=CARTESIAN_POINT('Ctrl Pts',(-0.674264766014723,0.850659477558785,
7.4499972894827));
#10749=CARTESIAN_POINT('Ctrl Pts',(-1.0215282433438,0.360895066694614,7.47433816416247));
#10750=CARTESIAN_POINT('Ctrl Pts',(-1.05495989572618,-0.237418239847793,
7.49863351661875));
#10751=CARTESIAN_POINT('Ctrl Pts',(-0.765493965690148,-0.760837611247353,
7.52288328690495));
#10752=CARTESIAN_POINT('Ctrl Pts',(-0.242921801622797,-1.0494710437018,
7.54708703215697));
#10753=CARTESIAN_POINT('Ctrl Pts',(0.351970225278986,-1.01590502989561,
7.57124451032626));
#10754=CARTESIAN_POINT('Ctrl Pts',(0.836883375362913,-0.67164669764715,
7.59535542482914));
#10755=CARTESIAN_POINT('Ctrl Pts',(1.06386470149691,-0.123233424848443,
7.61941953772808));
#10756=CARTESIAN_POINT('Ctrl Pts',(0.96448818932038,0.460735663933303,7.64343662004129));
#10757=CARTESIAN_POINT('Ctrl Pts',(0.570400865876502,0.901456165300417,
7.66740647649098));
#10758=CARTESIAN_POINT('Ctrl Pts',(0.00343128420266171,1.06462402223465,
7.69132893385857));
#10759=CARTESIAN_POINT('Ctrl Pts',(-0.562462013634023,0.901470864308901,
7.71520384653006));
#10760=CARTESIAN_POINT('Ctrl Pts',(-0.93920407838125,0.479325471899194,
7.73814860418777));
#10761=CARTESIAN_POINT('Ctrl Pts',(-1.04563381734369,-0.0487591387118346,
7.76016910772723));
#10762=CARTESIAN_POINT('Ctrl Pts',(-0.893388715718348,-0.541954927211641,
7.78127102299369));
#10763=CARTESIAN_POINT('Ctrl Pts',(-0.524509993111373,-0.901534190695079,
7.80233509266462));
#10764=CARTESIAN_POINT('Ctrl Pts',(-0.0292887386476584,-1.04113014278304,
7.82336134357856));
#10765=CARTESIAN_POINT('Ctrl Pts',(0.470719775145307,-0.926199174985292,
7.84434971997527));
#10766=CARTESIAN_POINT('Ctrl Pts',(0.920151044870203,-0.531393688850765,
7.86879213004602));
#10767=CARTESIAN_POINT('Ctrl Pts',(1.07869587043031,0.159420004343398,7.89666351654933));
#10768=CARTESIAN_POINT('Ctrl Pts',(0.723895499075924,0.770663707163572,
7.92445965347429));
#10769=CARTESIAN_POINT('Ctrl Pts',(0.182030232236923,1.01363048371111,7.948726105815));
#10770=CARTESIAN_POINT('Ctrl Pts',(-0.324136171745627,0.975741615999532,
7.96948836497335));
#10771=CARTESIAN_POINT('Ctrl Pts',(-0.714453631350278,0.723213312087363,
7.98848651554928));
#10772=CARTESIAN_POINT('Ctrl Pts',(-0.935497699150504,0.370852328564716,
8.00573022282306));
#10773=CARTESIAN_POINT('Ctrl Pts',(-1.00520551147936,0.003280843936954,
8.02122871265022));
#10774=CARTESIAN_POINT('Ctrl Pts',(-0.935399570902944,-0.363301629637604,
8.03670639912639));
#10775=CARTESIAN_POINT('Ctrl Pts',(-0.671741170896316,-0.785473331547596,
8.05731555952276));
#10776=CARTESIAN_POINT('Ctrl Pts',(-0.0835914591230814,-1.06937590558802,
8.08302618007272));
#10777=CARTESIAN_POINT('Ctrl Pts',(0.664820094277504,-0.838174757202306,
8.11379655253259));
#10778=CARTESIAN_POINT('Ctrl Pts',(1.05441848069546,-0.161982020970417,
8.14448592141602));
#10779=CARTESIAN_POINT('Ctrl Pts',(0.881123855699413,0.596820461156313,
8.17509503429765));
#10780=CARTESIAN_POINT('Ctrl Pts',(0.238762774028777,1.03430920701819,8.20562474600236));
#10781=CARTESIAN_POINT('Ctrl Pts',(-0.440989874038897,0.930485897466661,
8.23269309303528));
#10782=CARTESIAN_POINT('Ctrl Pts',(-0.854200921270452,0.525410375048001,
8.25632711980103));
#10783=CARTESIAN_POINT('Ctrl Pts',(-1.00008100917318,0.0531416845693213,
8.27655112488305));
#10784=CARTESIAN_POINT('Ctrl Pts',(-0.90200349917642,-0.431042585830742,
8.29674152510973));
#10785=CARTESIAN_POINT('Ctrl Pts',(-0.585232908856582,-0.808836535644948,
8.31689817148631));
#10786=CARTESIAN_POINT('Ctrl Pts',(-0.241484208369084,-0.943331975688694,
8.33199166132556));
#10787=CARTESIAN_POINT('Ctrl Pts',(-0.00313258390604597,-0.958028426645384,
8.34204308984535));
#10788=CARTESIAN_POINT('Ctrl Pts',(0.155630995470786,-0.948146354918541,
8.34874143218627));
#10789=CARTESIAN_POINT('Ctrl Pts',(0.388406644952516,-0.889043212840594,
8.35878305450209));
#10790=CARTESIAN_POINT('Ctrl Pts',(0.660946080093702,-0.717199923829581,
8.37215894305961));
#10791=CARTESIAN_POINT('Ctrl Pts',(0.949982129920854,-0.328582950010552,
8.39219849402223));
#10792=CARTESIAN_POINT('Ctrl Pts',(0.998559015277984,0.304265589788258,
8.41720373230134));
#10793=CARTESIAN_POINT('Ctrl Pts',(0.522077893834886,0.900628246456589,
8.44714268357634));
#10794=CARTESIAN_POINT('Ctrl Pts',(-0.165513598662709,1.00284693060682,
8.4745244155206));
#10795=CARTESIAN_POINT('Ctrl Pts',(-0.701855624130506,0.705135890791863,
8.49936815983874));
#10796=CARTESIAN_POINT('Ctrl Pts',(-0.967948575818185,0.223795924594876,
8.52169152062583));
#10797=CARTESIAN_POINT('Ctrl Pts',(-0.93711414110698,-0.325536385888489,
8.54397906340804));
#10798=CARTESIAN_POINT('Ctrl Pts',(-0.67803860118516,-0.6895070937393,8.56211163922283));
#10799=CARTESIAN_POINT('Ctrl Pts',(-0.325363913511247,-0.905040920367593,
8.57939955057773));
#10800=CARTESIAN_POINT('Ctrl Pts',(0.0309053846454797,-0.967971730440252,
8.59420275005887));
#10801=CARTESIAN_POINT('Ctrl Pts',(0.413941925614915,-0.864842868973118,
8.61063250335662));
#10802=CARTESIAN_POINT('Ctrl Pts',(0.700715405917063,-0.653424071291302,
8.62540408573038));
#10803=CARTESIAN_POINT('Ctrl Pts',(0.890003605091469,-0.351808044165019,
8.64016247285312));
#10804=CARTESIAN_POINT('Ctrl Pts',(0.967542406534895,0.0559962531859067,
8.65736364651605));
#10805=CARTESIAN_POINT('Ctrl Pts',(0.833760313033866,0.521285133638719,
8.67700070139823));
#10806=CARTESIAN_POINT('Ctrl Pts',(0.42782549810846,0.883792680066817,8.69906186563957));
#10807=CARTESIAN_POINT('Ctrl Pts',(-0.107804311833239,0.974704985814576,
8.72109429595876));
#10808=CARTESIAN_POINT('Ctrl Pts',(-0.609174652584766,0.766947011662965,
8.7430985571953));
#10809=CARTESIAN_POINT('Ctrl Pts',(-0.922729261913642,0.324844912449117,
8.76507576134807));
#10810=CARTESIAN_POINT('Ctrl Pts',(-0.952999507734519,-0.215677498529127,
8.78702678544552));
#10811=CARTESIAN_POINT('Ctrl Pts',(-0.691348090308507,-0.688911833502101,
8.80895262586299));
#10812=CARTESIAN_POINT('Ctrl Pts',(-0.218553588797013,-0.950119550572946,
8.83085424324479));
#10813=CARTESIAN_POINT('Ctrl Pts',(0.32017377908378,-0.919784087573411,
8.85273263486959));
#10814=CARTESIAN_POINT('Ctrl Pts',(0.759744995635515,-0.607799082156627,
8.87458879663461));
#10815=CARTESIAN_POINT('Ctrl Pts',(0.965755577871433,-0.11025296341866,
8.89642374112683));
#10816=CARTESIAN_POINT('Ctrl Pts',(0.875579662109175,0.420143968732924,
8.91823850470675));
#10817=CARTESIAN_POINT('Ctrl Pts',(0.517338405956845,0.820918470026088,
8.94003411305096));
#10818=CARTESIAN_POINT('Ctrl Pts',(0.0012710543841073,0.969544978443646,
8.96181165944999));
#10819=CARTESIAN_POINT('Ctrl Pts',(-0.514464942965089,0.820953664757525,
8.98357213567796));
#10820=CARTESIAN_POINT('Ctrl Pts',(-0.858337283734613,0.435843869483925,
9.00451148214707));
#10821=CARTESIAN_POINT('Ctrl Pts',(-0.955560714905759,-0.0466269226500807,
9.02463212714799));
#10822=CARTESIAN_POINT('Ctrl Pts',(-0.816688402207661,-0.497728249872681,
9.04393592539421));
#10823=CARTESIAN_POINT('Ctrl Pts',(-0.506889147550573,-0.799878736533962,
9.06162207865932));
#10824=CARTESIAN_POINT('Ctrl Pts',(-0.14096336145598,-0.927213398264503,
9.07769385094099));
#10825=CARTESIAN_POINT('Ctrl Pts',(0.324512190886538,-0.911102185093492,
9.09697223469682));
#10826=CARTESIAN_POINT('Ctrl Pts',(0.728968813708346,-0.636669415745461,
9.11624302783002));
#10827=CARTESIAN_POINT('Ctrl Pts',(0.91324192523573,-0.2091896101292,9.13550450393053));
#10828=CARTESIAN_POINT('Ctrl Pts',(0.932302842350122,0.254831083543151,
9.15476058856452));
#10829=CARTESIAN_POINT('Ctrl Pts',(0.626900263580331,0.785504982864274,
9.17882483506651));
#10830=CARTESIAN_POINT('Ctrl Pts',(0.0423452694845425,0.964740415964174,
9.20287985836102));
#10831=CARTESIAN_POINT('Ctrl Pts',(-0.405906098755213,0.843205768511259,
9.22211803373898));
#10832=CARTESIAN_POINT('Ctrl Pts',(-0.717235768498481,0.614120703650391,
9.23814771688336));
#10833=CARTESIAN_POINT('Ctrl Pts',(-0.92370760684931,0.235266265275963,
9.25578020037257));
#10834=CARTESIAN_POINT('Ctrl Pts',(-0.923376422631151,-0.235005878724949,
9.27501174354034));
#10835=CARTESIAN_POINT('Ctrl Pts',(-0.698715298937986,-0.648292214447006,
9.29424327143548));
#10836=CARTESIAN_POINT('Ctrl Pts',(-0.303406202904001,-0.903192481821634,
9.31347490228703));
#10837=CARTESIAN_POINT('Ctrl Pts',(0.16559811215366,-0.938655265798546,
9.33270600943893));
#10838=CARTESIAN_POINT('Ctrl Pts',(0.491608636905682,-0.791338058660878,
9.34733350869031));
#10839=CARTESIAN_POINT('Ctrl Pts',(0.666820161878111,-0.630086196708776,
9.35735100901671));
#10840=CARTESIAN_POINT('Ctrl Pts',(0.775546109169976,-0.497595093735688,
9.3645640119917));
#10841=CARTESIAN_POINT('Ctrl Pts',(0.914746049094079,-0.229100519953174,
9.37718769779949));
#10842=CARTESIAN_POINT('Ctrl Pts',(0.934696371728414,0.12593490391397,9.3916192338851));
#10843=CARTESIAN_POINT('Ctrl Pts',(0.810930047844375,0.448675148178548,
9.4060507946647));
#10844=CARTESIAN_POINT('Ctrl Pts',(0.603540213098328,0.725122428597784,
9.42048450263819));
#10845=CARTESIAN_POINT('Ctrl Pts',(0.214205829944543,0.940615684273133,
9.43853221348709));
#10846=CARTESIAN_POINT('Ctrl Pts',(-0.31933594831027,0.910615224040587,
9.460195939325));
#10847=CARTESIAN_POINT('Ctrl Pts',(-0.755217739844288,0.601392195346104,
9.48186844163729));
#10848=CARTESIAN_POINT('Ctrl Pts',(-0.959902232150957,0.10736858445662,
9.50355036655641));
#10849=CARTESIAN_POINT('Ctrl Pts',(-0.870316378158485,-0.420063150575497,
9.52524306057417));
#10850=CARTESIAN_POINT('Ctrl Pts',(-0.51366548932194,-0.819226222680466,
9.54694754310527));
#10851=CARTESIAN_POINT('Ctrl Pts',(0.00099722262819886,-0.967543954202361,
9.56866494808632));
#10852=CARTESIAN_POINT('Ctrl Pts',(0.516016920582239,-0.81922256521234,
9.5903963601957));
#10853=CARTESIAN_POINT('Ctrl Pts',(0.873436814265292,-0.419352238605789,
9.61214286014485));
#10854=CARTESIAN_POINT('Ctrl Pts',(0.963398958340639,0.10977813142819,9.63390552377525));
#10855=CARTESIAN_POINT('Ctrl Pts',(0.757897894439999,0.606061766756622,
9.65568540741735));
#10856=CARTESIAN_POINT('Ctrl Pts',(0.319489023351443,0.9172073481515,9.67748356901533));
#10857=CARTESIAN_POINT('Ctrl Pts',(-0.217739692090491,0.947441559483756,
9.69930104654587));
#10858=CARTESIAN_POINT('Ctrl Pts',(-0.689154860322401,0.686979141731466,
9.72113887780304));
#10859=CARTESIAN_POINT('Ctrl Pts',(-0.950001674292135,0.215160715023784,
9.74299805428903));
#10860=CARTESIAN_POINT('Ctrl Pts',(-0.919826616460147,-0.323661293630411,
9.76487966279437));
#10861=CARTESIAN_POINT('Ctrl Pts',(-0.607283029397313,-0.764355668580401,
9.78678450836089));
#10862=CARTESIAN_POINT('Ctrl Pts',(-0.107654549029002,-0.971392889114284,
9.80871400622512));
#10863=CARTESIAN_POINT('Ctrl Pts',(0.426152293844201,-0.880962937933544,
9.8306681505383));
#10864=CARTESIAN_POINT('Ctrl Pts',(0.830424803659154,-0.519624647538494,
9.85265006399591));
#10865=CARTESIAN_POINT('Ctrl Pts',(0.930600595159381,-0.172510125317866,
9.86731890233875));
#10866=CARTESIAN_POINT('Ctrl Pts',(0.930624104877249,0.00212604796771284,
9.87466239594617));
#10867=CARTESIAN_POINT('Ctrl Pts',(1.08384642846031,-0.000793256800902784,
7.29413292869025));
#10868=CARTESIAN_POINT('Ctrl Pts',(1.08381908929503,0.202289003082833,7.30267258708788));
#10869=CARTESIAN_POINT('Ctrl Pts',(0.967159117688111,0.606890912023917,
7.31977033977986));
#10870=CARTESIAN_POINT('Ctrl Pts',(0.495930087867846,1.02807430064273,7.34539171275669));
#10871=CARTESIAN_POINT('Ctrl Pts',(-0.126761042383259,1.13367938470921,
7.37100435156813));
#10872=CARTESIAN_POINT('Ctrl Pts',(-0.709971284708507,0.892049379954826,
7.39660097985035));
#10873=CARTESIAN_POINT('Ctrl Pts',(-1.07501405252591,0.377418129162179,
7.42218333959883));
#10874=CARTESIAN_POINT('Ctrl Pts',(-1.11030586598071,-0.252127576999562,
7.4477491320311));
#10875=CARTESIAN_POINT('Ctrl Pts',(-0.805456401016912,-0.803593486480699,
7.47329786737596));
#10876=CARTESIAN_POINT('Ctrl Pts',(-0.254335423454531,-1.10811832577815,
7.4988282519598));
#10877=CARTESIAN_POINT('Ctrl Pts',(0.373850028247498,-1.07277814526268,
7.52433935505151));
#10878=CARTESIAN_POINT('Ctrl Pts',(0.886537206986384,-0.708926672984277,
7.54983010396061));
#10879=CARTESIAN_POINT('Ctrl Pts',(1.12684930546936,-0.128563840777488,
7.57529949924907));
#10880=CARTESIAN_POINT('Ctrl Pts',(1.02165804861735,0.490150925268269,7.6007465283239));
#10881=CARTESIAN_POINT('Ctrl Pts',(0.603764038088763,0.957636470965819,
7.62617019061896));
#10882=CARTESIAN_POINT('Ctrl Pts',(0.00185210167093897,1.13095496972185,
7.65156953889001));
#10883=CARTESIAN_POINT('Ctrl Pts',(-0.59956549271009,0.9576526886088,7.67694353645162));
#10884=CARTESIAN_POINT('Ctrl Pts',(-1.00039059858681,0.508644588622468,
7.70135260850433));
#10885=CARTESIAN_POINT('Ctrl Pts',(-1.11376643951718,-0.0535942367798588,
7.72479874105888));
#10886=CARTESIAN_POINT('Ctrl Pts',(-0.951594070937359,-0.579139877751677,
7.74728507022348));
#10887=CARTESIAN_POINT('Ctrl Pts',(-0.558264880040219,-0.962633038967035,
7.76974846765362));
#10888=CARTESIAN_POINT('Ctrl Pts',(-0.0297845563498375,-1.11165847490554,
7.79218801827507));
#10889=CARTESIAN_POINT('Ctrl Pts',(0.504224144516551,-0.988964719556773,
7.8146035994472));
#10890=CARTESIAN_POINT('Ctrl Pts',(0.984577474321374,-0.56707344670203,
7.84072646125844));
#10891=CARTESIAN_POINT('Ctrl Pts',(1.15430617570018,0.171814819585418,7.87054013838732));
#10892=CARTESIAN_POINT('Ctrl Pts',(0.774547719067364,0.826325866763944,
7.90030160483131));
#10893=CARTESIAN_POINT('Ctrl Pts',(0.193979612614955,1.08670118860458,7.9263023705649));
#10894=CARTESIAN_POINT('Ctrl Pts',(-0.348665393370604,1.04611990516275,
7.94856102173379));
#10895=CARTESIAN_POINT('Ctrl Pts',(-0.767359045720052,0.775275157221321,
7.9689396492515));
#10896=CARTESIAN_POINT('Ctrl Pts',(-1.00458183390253,0.397155764877826,
7.98744444059531));
#10897=CARTESIAN_POINT('Ctrl Pts',(-1.07942987205928,0.00256356478130836,
8.00408248537729));
#10898=CARTESIAN_POINT('Ctrl Pts',(-1.0044783210053,-0.391111487886477,
8.02070397667786));
#10899=CARTESIAN_POINT('Ctrl Pts',(-0.721260789217433,-0.844639481874048,
8.04284350578955));
#10900=CARTESIAN_POINT('Ctrl Pts',(-0.0891736393931901,-1.14984162670411,
8.0704763974833));
#10901=CARTESIAN_POINT('Ctrl Pts',(0.715678720844839,-0.901299501303157,
8.1035658986358));
#10902=CARTESIAN_POINT('Ctrl Pts',(1.13492007912664,-0.17381149421113,8.13658458374464));
#10903=CARTESIAN_POINT('Ctrl Pts',(0.948455032144445,0.64295968933924,8.16953075755057));
#10904=CARTESIAN_POINT('Ctrl Pts',(0.256816826853416,1.11407722004625,8.20240312942989));
#10905=CARTESIAN_POINT('Ctrl Pts',(-0.475327032992583,1.00229310544698,
8.23155630552289));
#10906=CARTESIAN_POINT('Ctrl Pts',(-0.920474247117944,0.565929865334376,
8.25701571321748));
#10907=CARTESIAN_POINT('Ctrl Pts',(-1.07765167819056,0.0571232220460662,
8.27880380868564));
#10908=CARTESIAN_POINT('Ctrl Pts',(-0.971985175738061,-0.464564051003078,
8.30055729936963));
#10909=CARTESIAN_POINT('Ctrl Pts',(-0.630665261642236,-0.871644705172118,
8.32227584244456));
#10910=CARTESIAN_POINT('Ctrl Pts',(-0.260275322606424,-1.01656300716899,
8.33853832228072));
#10911=CARTESIAN_POINT('Ctrl Pts',(-0.00344558452418022,-1.0323993719803,
8.34936892151002));
#10912=CARTESIAN_POINT('Ctrl Pts',(0.167623965316464,-1.02175149523021,
8.35658635286812));
#10913=CARTESIAN_POINT('Ctrl Pts',(0.418436678562632,-0.958069044630896,
8.36740579432199));
#10914=CARTESIAN_POINT('Ctrl Pts',(0.712079660427613,-0.7729198568326,8.3818167331061));
#10915=CARTESIAN_POINT('Ctrl Pts',(1.02347973785374,-0.354227798098456,
8.40340626006335));
#10916=CARTESIAN_POINT('Ctrl Pts',(1.07578845759894,0.327516652661325,8.43034229555736));
#10917=CARTESIAN_POINT('Ctrl Pts',(0.562588863844005,0.969761430420295,
8.46258290726966));
#10918=CARTESIAN_POINT('Ctrl Pts',(-0.177715492101827,1.07977400632615,
8.49206088659617));
#10919=CARTESIAN_POINT('Ctrl Pts',(-0.754969512302287,0.759321620849947,
8.51879847856748));
#10920=CARTESIAN_POINT('Ctrl Pts',(-1.04125073281678,0.241419209252838,
8.54281498297182));
#10921=CARTESIAN_POINT('Ctrl Pts',(-1.00805722180633,-0.349404771948186,
8.56678423739501));
#10922=CARTESIAN_POINT('Ctrl Pts',(-0.729517853526143,-0.740677351451125,
8.58627564980444));
#10923=CARTESIAN_POINT('Ctrl Pts',(-0.350480132340932,-0.972316810663511,
8.60485496723001));
#10924=CARTESIAN_POINT('Ctrl Pts',(0.0322991958263789,-1.03990993998121,
8.62075891439363));
#10925=CARTESIAN_POINT('Ctrl Pts',(0.443650471011225,-0.929143712575293,
8.63840200647036));
#10926=CARTESIAN_POINT('Ctrl Pts',(0.751518738327972,-0.702159843963306,
8.6542599534087));
#10927=CARTESIAN_POINT('Ctrl Pts',(0.954636456966557,-0.37848104417437,
8.67009604620781));
#10928=CARTESIAN_POINT('Ctrl Pts',(1.03779888771484,0.0589833027264458,
8.68854704443214));
#10929=CARTESIAN_POINT('Ctrl Pts',(0.894321819630977,0.557814720788599,
8.7095975416509));
#10930=CARTESIAN_POINT('Ctrl Pts',(0.459360346577918,0.946166909345621,
8.73323177261074));
#10931=CARTESIAN_POINT('Ctrl Pts',(-0.114118824404391,1.04344007211952,
8.75681788745377));
#10932=CARTESIAN_POINT('Ctrl Pts',(-0.650476848794739,0.82111535279448,
8.78035613912247));
#10933=CARTESIAN_POINT('Ctrl Pts',(-0.985604987995532,0.348480992052307,
8.80384648245865));
#10934=CARTESIAN_POINT('Ctrl Pts',(-1.01786740958942,-0.228839867930964,
8.82728905034341));
#10935=CARTESIAN_POINT('Ctrl Pts',(-0.738589557901741,-0.733806334779716,
8.85068393868067));
#10936=CARTESIAN_POINT('Ctrl Pts',(-0.234488932120026,-1.01222446231625,
8.87403130042571));
#10937=CARTESIAN_POINT('Ctrl Pts',(0.339309874015096,-0.979835882831324,
8.89733130405925));
#10938=CARTESIAN_POINT('Ctrl Pts',(0.806983157414378,-0.647805656061189,
8.920584146721));
#10939=CARTESIAN_POINT('Ctrl Pts',(1.02587940738221,-0.11891857779353,8.94379005403647));
#10940=CARTESIAN_POINT('Ctrl Pts',(0.930047505375005,0.444228970333776,
8.9669492663554));
#10941=CARTESIAN_POINT('Ctrl Pts',(0.550037348365757,0.869224147485282,
8.99006207126683));
#10942=CARTESIAN_POINT('Ctrl Pts',(0.00331688177892927,1.02658582996463,
9.01312872078293));
#10943=CARTESIAN_POINT('Ctrl Pts',(-0.542345277424951,0.869275726604705,
9.03614961115852));
#10944=CARTESIAN_POINT('Ctrl Pts',(-0.905667395299237,0.4622482747292,9.05827393317691));
#10945=CARTESIAN_POINT('Ctrl Pts',(-1.00821264225331,-0.047010260451699,
9.07950822199612));
#10946=CARTESIAN_POINT('Ctrl Pts',(-0.861732962585674,-0.522594137999902,
9.09985879309251));
#10947=CARTESIAN_POINT('Ctrl Pts',(-0.535452731740728,-0.840721246165385,
9.11848100566275));
#10948=CARTESIAN_POINT('Ctrl Pts',(-0.150527266233238,-0.974636173165108,
9.13538461085382));
#10949=CARTESIAN_POINT('Ctrl Pts',(0.338682804184835,-0.957648390576258,
9.15564420037776));
#10950=CARTESIAN_POINT('Ctrl Pts',(0.76304477781549,-0.669506770040774,
9.1758634753981));
#10951=CARTESIAN_POINT('Ctrl Pts',(0.956095920089128,-0.221513534188684,
9.19604620427903));
#10952=CARTESIAN_POINT('Ctrl Pts',(0.976011877017348,0.26431211473213,9.2162043883441));
#10953=CARTESIAN_POINT('Ctrl Pts',(0.656548774825726,0.81891683061587,9.24135284185631));
#10954=CARTESIAN_POINT('Ctrl Pts',(0.0466882531800841,1.00566644796459,
9.26644056558201));
#10955=CARTESIAN_POINT('Ctrl Pts',(-0.420196777981749,0.879028902672049,
9.28647688240236));
#10956=CARTESIAN_POINT('Ctrl Pts',(-0.744120699223029,0.640630339035476,
9.30315438470658));
#10957=CARTESIAN_POINT('Ctrl Pts',(-0.95861694874501,0.246913067796348,
9.32147257780598));
#10958=CARTESIAN_POINT('Ctrl Pts',(-0.958178271491326,-0.241092352278578,
9.3414279620528));
#10959=CARTESIAN_POINT('Ctrl Pts',(-0.725325955917838,-0.669287711537651,
9.361352107215));
#10960=CARTESIAN_POINT('Ctrl Pts',(-0.31628593978967,-0.932926599228729,
9.3812463447098));
#10961=CARTESIAN_POINT('Ctrl Pts',(0.168249973887814,-0.969479581836067,
9.40111282491626));
#10962=CARTESIAN_POINT('Ctrl Pts',(0.504451373670123,-0.817462569521572,
9.4161945546897));
#10963=CARTESIAN_POINT('Ctrl Pts',(0.685009996862284,-0.6512836464409,9.42651766084202));
#10964=CARTESIAN_POINT('Ctrl Pts',(0.797005370990673,-0.514805420344457,
9.43394717676915));
#10965=CARTESIAN_POINT('Ctrl Pts',(0.940278681951758,-0.23840503025821,
9.44694090738106));
#10966=CARTESIAN_POINT('Ctrl Pts',(0.960696404399766,0.126535341586046,
9.46177038655293));
#10967=CARTESIAN_POINT('Ctrl Pts',(0.833607413309956,0.457875833720658,
9.47658602820858));
#10968=CARTESIAN_POINT('Ctrl Pts',(0.620852271531433,0.741434358704751,
9.49139014459053));
#10969=CARTESIAN_POINT('Ctrl Pts',(0.221996454884777,0.962065864953804,
9.50987237532345));
#10970=CARTESIAN_POINT('Ctrl Pts',(-0.323541174854107,0.931248882602088,
9.53201979030854));
#10971=CARTESIAN_POINT('Ctrl Pts',(-0.768333094902132,0.615525665216968,
9.55413527108079));
#10972=CARTESIAN_POINT('Ctrl Pts',(-0.976727100725712,0.112174129761956,
9.5762202682564));
#10973=CARTESIAN_POINT('Ctrl Pts',(-0.885486082363011,-0.424142120536936,
9.59827535662572));
#10974=CARTESIAN_POINT('Ctrl Pts',(-0.523378588106049,-0.829197320524031,
9.62030154695759));
#10975=CARTESIAN_POINT('Ctrl Pts',(-0.0019324619193897,-0.979320702375544,
9.64229967474914));
#10976=CARTESIAN_POINT('Ctrl Pts',(0.518815530859397,-0.829199944725929,
9.66427069811794));
#10977=CARTESIAN_POINT('Ctrl Pts',(0.87944912287424,-0.425517469831924,
9.68621553547096));
#10978=CARTESIAN_POINT('Ctrl Pts',(0.969932314485265,0.107543910523038,
9.70813515474387));
#10979=CARTESIAN_POINT('Ctrl Pts',(0.763171810925342,0.606487765894584,
9.73003051320366));
#10980=CARTESIAN_POINT('Ctrl Pts',(0.323116327168651,0.918622711733031,
9.75190260774064));
#10981=CARTESIAN_POINT('Ctrl Pts',(-0.215009582857648,0.948761113833324,
9.77375241361181));
#10982=CARTESIAN_POINT('Ctrl Pts',(-0.686236351315572,0.688237658598508,
9.79558097984185));
#10983=CARTESIAN_POINT('Ctrl Pts',(-0.946396968696602,0.217366324799682,
9.81738921471157));
#10984=CARTESIAN_POINT('Ctrl Pts',(-0.916205377388286,-0.319261288483713,
9.83917839754132));
#10985=CARTESIAN_POINT('Ctrl Pts',(-0.605414027709865,-0.757254947166093,
9.86094896999974));
#10986=CARTESIAN_POINT('Ctrl Pts',(-0.109657320635582,-0.962534333662517,
9.88270327490055));
#10987=CARTESIAN_POINT('Ctrl Pts',(0.418914924439416,-0.872861288741235,
9.90443938873523));
#10988=CARTESIAN_POINT('Ctrl Pts',(0.818388829673488,-0.51557521947165,
9.92616491491646));
#10989=CARTESIAN_POINT('Ctrl Pts',(0.917073865342883,-0.173169092744639,
9.94062996432396));
#10990=CARTESIAN_POINT('Ctrl Pts',(0.917097049589342,-0.000950604005939382,
9.94787179370752));
#10991=CARTESIAN_POINT('Ctrl Pts',(1.0670179066401,0.00225746580351556,
7.22152958911222));
#10992=CARTESIAN_POINT('Ctrl Pts',(1.06699097611627,0.202304233294702,7.2299416043168));
#10993=CARTESIAN_POINT('Ctrl Pts',(0.952169493387724,0.600953273779197,
7.24678378615139));
#10994=CARTESIAN_POINT('Ctrl Pts',(0.487186394855587,1.01678373272383,7.27207042045906));
#10995=CARTESIAN_POINT('Ctrl Pts',(-0.128346163220755,1.12129993252972,
7.29738651367873));
#10996=CARTESIAN_POINT('Ctrl Pts',(-0.705870567011168,0.882175433229343,
7.32272911076493));
#10997=CARTESIAN_POINT('Ctrl Pts',(-1.0680195677792,0.371849003294253,7.34809819670836));
#10998=CARTESIAN_POINT('Ctrl Pts',(-1.10321422557632,-0.253530752930648,
7.37349240932164));
#10999=CARTESIAN_POINT('Ctrl Pts',(-0.800005714726182,-0.802315846496021,
7.39891096663443));
#11000=CARTESIAN_POINT('Ctrl Pts',(-0.250806475805171,-1.10594008465963,
7.42435280627046));
#11001=CARTESIAN_POINT('Ctrl Pts',(0.376295106921614,-1.07080374820359,
7.4498169663272));
#11002=CARTESIAN_POINT('Ctrl Pts',(0.889008624586151,-0.707108832454598,
7.47530242608526));
#11003=CARTESIAN_POINT('Ctrl Pts',(1.12981834509025,-0.125917689478273,
7.50080817431521));
#11004=CARTESIAN_POINT('Ctrl Pts',(1.02443603606273,0.494773142194464,7.52633316714341));
#11005=CARTESIAN_POINT('Ctrl Pts',(0.604646428898813,0.964593536017731,
7.55187637605968));
#11006=CARTESIAN_POINT('Ctrl Pts',(-0.00109375463389684,1.13916272997907,
7.57743671976539));
#11007=CARTESIAN_POINT('Ctrl Pts',(-0.607399194221062,0.964601513127144,
7.60301318476041));
#11008=CARTESIAN_POINT('Ctrl Pts',(-1.01221199749175,0.511330398063977,
7.62765674322727));
#11009=CARTESIAN_POINT('Ctrl Pts',(-1.12696398058896,-0.0572091674480348,
7.65136486655048));
#11010=CARTESIAN_POINT('Ctrl Pts',(-0.962827544625284,-0.589451999852308,
7.67413480745332));
#11011=CARTESIAN_POINT('Ctrl Pts',(-0.56400406423614,-0.978430974917163,
7.69691430442555));
#11012=CARTESIAN_POINT('Ctrl Pts',(-0.0273139330862592,-1.12987903202044,
7.71970276832014));
#11013=CARTESIAN_POINT('Ctrl Pts',(0.515815112770866,-1.00518016474251,
7.74249910058463));
#11014=CARTESIAN_POINT('Ctrl Pts',(1.00510855649337,-0.575600695245217,
7.76910313379358));
#11015=CARTESIAN_POINT('Ctrl Pts',(1.17855810364818,0.178171254926354,7.79951779751799));
#11016=CARTESIAN_POINT('Ctrl Pts',(0.790555243745666,0.847481198951724,
7.82994286951095));
#11017=CARTESIAN_POINT('Ctrl Pts',(0.195989759376802,1.11426017821105,7.85657119093045));
#11018=CARTESIAN_POINT('Ctrl Pts',(-0.360542451510464,1.072730591672,7.87939875619507));
#11019=CARTESIAN_POINT('Ctrl Pts',(-0.790575610104427,0.794655665848824,
7.90032600950703));
#11020=CARTESIAN_POINT('Ctrl Pts',(-1.03452330807482,0.405894124045869,
7.91935211503271));
#11021=CARTESIAN_POINT('Ctrl Pts',(-1.11159730313937,-0.000226215064824152,
7.93647617919723));
#11022=CARTESIAN_POINT('Ctrl Pts',(-1.03440926459159,-0.405828742159562,
7.95360049379582));
#11023=CARTESIAN_POINT('Ctrl Pts',(-0.74237760663053,-0.87357549827158,
7.97643284086373));
#11024=CARTESIAN_POINT('Ctrl Pts',(-0.0896511524093107,-1.18902475277104,
8.00497202233576));
#11025=CARTESIAN_POINT('Ctrl Pts',(0.743363174455746,-0.932124406438126,
8.03921482596584));
#11026=CARTESIAN_POINT('Ctrl Pts',(1.17833662686497,-0.177955302960707,
8.0734505711755));
#11027=CARTESIAN_POINT('Ctrl Pts',(0.984923832475398,0.670619764075562,
8.10767668130492));
#11028=CARTESIAN_POINT('Ctrl Pts',(0.265230218108454,1.16122051794983,8.14189039895527));
#11029=CARTESIAN_POINT('Ctrl Pts',(-0.498244706977025,1.04490742079478,
8.17228939848879));
#11030=CARTESIAN_POINT('Ctrl Pts',(-0.96319243578791,0.589275579142102,
8.19887688574252));
#11031=CARTESIAN_POINT('Ctrl Pts',(-1.1276004842514,0.0573158710798558,
8.22165762197572));
#11032=CARTESIAN_POINT('Ctrl Pts',(-1.01706918705279,-0.488791893957402,
8.24442896924834));
#11033=CARTESIAN_POINT('Ctrl Pts',(-0.65942985328418,-0.9154574609399,8.26718997588247));
#11034=CARTESIAN_POINT('Ctrl Pts',(-0.270837562173685,-1.06755876416323,
8.28425279203188));
#11035=CARTESIAN_POINT('Ctrl Pts',(-0.00118687354693406,-1.08418781783305,
8.29562403461343));
#11036=CARTESIAN_POINT('Ctrl Pts',(0.17847181968188,-1.07300615066178,8.30320390908866));
#11037=CARTESIAN_POINT('Ctrl Pts',(0.441991001954779,-1.00610838488519,
8.31457153222276));
#11038=CARTESIAN_POINT('Ctrl Pts',(0.750736604364479,-0.811461732201089,
8.3297233770891));
#11039=CARTESIAN_POINT('Ctrl Pts',(1.07843616258299,-0.370936248534933,
8.35244115703416));
#11040=CARTESIAN_POINT('Ctrl Pts',(1.13374581637679,0.347265474782159,8.38081929419995));
#11041=CARTESIAN_POINT('Ctrl Pts',(0.592433182066138,1.02511972772588,8.41484104544098));
#11042=CARTESIAN_POINT('Ctrl Pts',(-0.189892820508684,1.14158783659837,
8.44599497305806));
#11043=CARTESIAN_POINT('Ctrl Pts',(-0.800772820980421,0.802593366402982,
8.47428867201138));
#11044=CARTESIAN_POINT('Ctrl Pts',(-1.10410464127913,0.254019264636482,
8.49973091044463));
#11045=CARTESIAN_POINT('Ctrl Pts',(-1.06899657652552,-0.372507568119275,
8.52514967281803));
#11046=CARTESIAN_POINT('Ctrl Pts',(-0.7733700537891,-0.787895550254676,
8.54584195730769));
#11047=CARTESIAN_POINT('Ctrl Pts',(-0.370740708663388,-1.03396781530568,
8.56557858405426));
#11048=CARTESIAN_POINT('Ctrl Pts',(0.036128362188144,-1.10585716589204,
8.58248423797523));
#11049=CARTESIAN_POINT('Ctrl Pts',(0.473720894744957,-0.988052361384637,
8.60125353364536));
#11050=CARTESIAN_POINT('Ctrl Pts',(0.80142920960278,-0.746466523315921,
8.61813325756913));
#11051=CARTESIAN_POINT('Ctrl Pts',(1.01778681299134,-0.401731344034236,
8.63500132881749));
#11052=CARTESIAN_POINT('Ctrl Pts',(1.10643741011627,0.0644691098389064,
8.65466549145617));
#11053=CARTESIAN_POINT('Ctrl Pts',(0.953481848200125,0.596494435383873,
8.67711832298153));
#11054=CARTESIAN_POINT('Ctrl Pts',(0.489254428552112,1.01107283728095,8.7023473450177));
#11055=CARTESIAN_POINT('Ctrl Pts',(-0.123357404494991,1.11505446266801,
8.72754575370462));
#11056=CARTESIAN_POINT('Ctrl Pts',(-0.696794985125646,0.877430464208332,
8.75271243011979));
#11057=CARTESIAN_POINT('Ctrl Pts',(-1.05539207302399,0.371804106734305,
8.77784666980832));
#11058=CARTESIAN_POINT('Ctrl Pts',(-1.08999120326104,-0.246294887366169,
8.80294760364296));
#11059=CARTESIAN_POINT('Ctrl Pts',(-0.790831476581851,-0.7873228005966,
8.82801445891056));
#11060=CARTESIAN_POINT('Ctrl Pts',(-0.250437283560287,-1.08584491695925,
8.85304644391363));
#11061=CARTESIAN_POINT('Ctrl Pts',(0.365074934754753,-1.05115032210123,
8.87804279858019));
#11062=CARTESIAN_POINT('Ctrl Pts',(0.867054606378142,-0.694819513608586,
8.90300278281863));
#11063=CARTESIAN_POINT('Ctrl Pts',(1.1021587421701,-0.126881195388152,8.92792567275981));
#11064=CARTESIAN_POINT('Ctrl Pts',(0.999234894086778,0.478167753869344,
8.95281077626079));
#11065=CARTESIAN_POINT('Ctrl Pts',(0.59079348095087,0.935010182874376,8.97765740192141));
#11066=CARTESIAN_POINT('Ctrl Pts',(0.00289559293650473,1.10425340130915,
9.00246494193154));
#11067=CARTESIAN_POINT('Ctrl Pts',(-0.58410289937492,0.935052600972256,
9.02723269116248));
#11068=CARTESIAN_POINT('Ctrl Pts',(-0.975094294651602,0.497057410139674,
9.05104442397967));
#11069=CARTESIAN_POINT('Ctrl Pts',(-1.08549188235095,-0.0511126263223194,
9.0739041956868));
#11070=CARTESIAN_POINT('Ctrl Pts',(-0.927797132691072,-0.563142626479479,
9.09581584631526));
#11071=CARTESIAN_POINT('Ctrl Pts',(-0.576444633511331,-0.905731153030661,
9.11587150880217));
#11072=CARTESIAN_POINT('Ctrl Pts',(-0.16186322904714,-1.04996464479364,
9.13407984159281));
#11073=CARTESIAN_POINT('Ctrl Pts',(0.365077377739307,-1.03167887835473,
9.15590342972986));
#11074=CARTESIAN_POINT('Ctrl Pts',(0.822261614921547,-0.721264636910472,
9.1776904595879));
#11075=CARTESIAN_POINT('Ctrl Pts',(1.03025713637287,-0.238612529479814,
9.199437337924));
#11076=CARTESIAN_POINT('Ctrl Pts',(1.05171274317535,0.284808676532102,9.22115764762888));
#11077=CARTESIAN_POINT('Ctrl Pts',(0.707499007137911,0.882392330252907,
9.24826137586986));
#11078=CARTESIAN_POINT('Ctrl Pts',(0.0503973500479551,1.08358547878404,
9.27529841784466));
#11079=CARTESIAN_POINT('Ctrl Pts',(-0.452565343899477,0.9471545860309,9.2968858692952));
#11080=CARTESIAN_POINT('Ctrl Pts',(-0.801496735835974,0.690347253274425,
9.31485263733184));
#11081=CARTESIAN_POINT('Ctrl Pts',(-1.03251942952317,0.266238466090755,
9.33458892725171));
#11082=CARTESIAN_POINT('Ctrl Pts',(-1.03204243532931,-0.259297874573609,
9.35608057654046));
#11083=CARTESIAN_POINT('Ctrl Pts',(-0.781296145011018,-0.720337835230956,
9.37753649325143));
#11084=CARTESIAN_POINT('Ctrl Pts',(-0.340960105513239,-1.00413521062253,
9.39895573092214));
#11085=CARTESIAN_POINT('Ctrl Pts',(0.18048440489374,-1.04344608683549,9.42033660154328));
#11086=CARTESIAN_POINT('Ctrl Pts',(0.542239509342812,-0.879875126181648,
9.43656964857728));
#11087=CARTESIAN_POINT('Ctrl Pts',(0.736445066942167,-0.70113509377245,
9.44767340469813));
#11088=CARTESIAN_POINT('Ctrl Pts',(0.856894738517867,-0.55435325618568,
9.45566431872803));
#11089=CARTESIAN_POINT('Ctrl Pts',(1.01096117719817,-0.257122260199454,
9.46963825282641));
#11090=CARTESIAN_POINT('Ctrl Pts',(1.03289239306723,0.135256216575748,9.48558750066562));
#11091=CARTESIAN_POINT('Ctrl Pts',(0.896311081511608,0.491323200624549,
9.50151009167922));
#11092=CARTESIAN_POINT('Ctrl Pts',(0.667724538317195,0.795974688107478,
9.51741707525718));
#11093=CARTESIAN_POINT('Ctrl Pts',(0.239306522759663,1.03291901978371,9.53727288403102));
#11094=CARTESIAN_POINT('Ctrl Pts',(-0.346296088438099,0.99979161701914,
9.56105101819272));
#11095=CARTESIAN_POINT('Ctrl Pts',(-0.82345191390219,0.661042061037232,
9.58478160219318));
#11096=CARTESIAN_POINT('Ctrl Pts',(-1.04683085355964,0.121359459090256,
9.60846407228079));
#11097=CARTESIAN_POINT('Ctrl Pts',(-0.94901887957637,-0.453248775549408,
9.6320986882585));
#11098=CARTESIAN_POINT('Ctrl Pts',(-0.561282561137808,-0.886881598782615,
9.65568536824822));
#11099=CARTESIAN_POINT('Ctrl Pts',(-0.00339911447116993,-1.0474281541931,
9.67922421242135));
#11100=CARTESIAN_POINT('Ctrl Pts',(0.553257143873196,-0.886885387621517,
9.7027152735699));
#11101=CARTESIAN_POINT('Ctrl Pts',(0.938395324818619,-0.455667215824606,
9.72615865946567));
#11102=CARTESIAN_POINT('Ctrl Pts',(1.03488266426865,0.113203951634057,9.74955449029365));
#11103=CARTESIAN_POINT('Ctrl Pts',(0.81437044505405,0.645134483473366,9.77290291527007));
#11104=CARTESIAN_POINT('Ctrl Pts',(0.345602036856306,0.977539014113442,
9.79620411104843));
#11105=CARTESIAN_POINT('Ctrl Pts',(-0.227009525616586,1.00952652784022,
9.81945827173785));
#11106=CARTESIAN_POINT('Ctrl Pts',(-0.727866299354974,0.732522380427292,
9.84266563594512));
#11107=CARTESIAN_POINT('Ctrl Pts',(-1.00402898230868,0.232497928985327,
9.86582641828462));
#11108=CARTESIAN_POINT('Ctrl Pts',(-0.971909096055521,-0.336665090315949,
9.8889409732355));
#11109=CARTESIAN_POINT('Ctrl Pts',(-0.642564620330116,-0.800621732870167,
9.91200940971414));
#11110=CARTESIAN_POINT('Ctrl Pts',(-0.117930823376944,-1.01775421835117,
9.93503245984089));
#11111=CARTESIAN_POINT('Ctrl Pts',(0.44070282986155,-0.92286732415585,9.95800952149167));
#11112=CARTESIAN_POINT('Ctrl Pts',(0.862306840760016,-0.545707449143151,
9.98094303612929));
#11113=CARTESIAN_POINT('Ctrl Pts',(0.966341550947047,-0.18465912338656,
9.99619919808942));
#11114=CARTESIAN_POINT('Ctrl Pts',(0.966365964358855,-0.00331008130675842,
10.0038249694641));
#11115=CARTESIAN_POINT('Ctrl Pts',(1.0224395231333,0.0031540044764207,7.20006622055264));
#11116=CARTESIAN_POINT('Ctrl Pts',(1.02241370724182,0.194920999938243,7.20813006933056));
#11117=CARTESIAN_POINT('Ctrl Pts',(0.912366886309143,0.576958392287561,
7.22427144136625));
#11118=CARTESIAN_POINT('Ctrl Pts',(0.466456717327568,0.975815803916186,
7.24852425219416));
#11119=CARTESIAN_POINT('Ctrl Pts',(-0.124217636317022,1.0761482596652,7.27281852486299));
#11120=CARTESIAN_POINT('Ctrl Pts',(-0.678781147637653,0.846597884923694,
7.29715370167105));
#11121=CARTESIAN_POINT('Ctrl Pts',(-1.0267885200925,0.356304901332808,7.32152945959023));
#11122=CARTESIAN_POINT('Ctrl Pts',(-1.0606890229609,-0.244950870661962,
7.34594534636892));
#11123=CARTESIAN_POINT('Ctrl Pts',(-0.769035493636253,-0.772955750304005,
7.3704009447994));
#11124=CARTESIAN_POINT('Ctrl Pts',(-0.240329864575481,-1.0653237085793,
7.39489579641338));
#11125=CARTESIAN_POINT('Ctrl Pts',(0.363839304010974,-1.03153783690531,
7.41942943142408));
#11126=CARTESIAN_POINT('Ctrl Pts',(0.858198998883183,-0.680943831755809,
7.44400135772063));
#11127=CARTESIAN_POINT('Ctrl Pts',(1.0906063677628,-0.120209327641914,7.46861106610192));
#11128=CARTESIAN_POINT('Ctrl Pts',(0.988919658857672,0.479131132259177,
7.49325801533902));
#11129=CARTESIAN_POINT('Ctrl Pts',(0.583314808696736,0.933183422390409,
7.51794166559975));
#11130=CARTESIAN_POINT('Ctrl Pts',(-0.00247975052802087,1.1020802294482,
7.54266141162343));
#11131=CARTESIAN_POINT('Ctrl Pts',(-0.589337810114969,0.933196369368626,
7.56741671884064));
#11132=CARTESIAN_POINT('Ctrl Pts',(-0.981531482742348,0.494164393687638,
7.59128867034107));
#11133=CARTESIAN_POINT('Ctrl Pts',(-1.09283525118144,-0.0570023695692098,
7.61427269700993));
#11134=CARTESIAN_POINT('Ctrl Pts',(-0.933642969752733,-0.573400485891667,
7.63636381653099));
#11135=CARTESIAN_POINT('Ctrl Pts',(-0.546444722767111,-0.95111688919212,
7.65848129757189));
#11136=CARTESIAN_POINT('Ctrl Pts',(-0.0249538254466607,-1.09833623866965,
7.68062474544456));
#11137=CARTESIAN_POINT('Ctrl Pts',(0.503244146713521,-0.977119473107213,
7.70279347292931));
#11138=CARTESIAN_POINT('Ctrl Pts',(0.979497658227209,-0.559085504295418,
7.72868549174814));
#11139=CARTESIAN_POINT('Ctrl Pts',(1.14865259980211,0.175228209374103,7.75831545469268));
#11140=CARTESIAN_POINT('Ctrl Pts',(0.770334243068627,0.828201516454482,
7.78799180006802));
#11141=CARTESIAN_POINT('Ctrl Pts',(0.18976680663554,1.0887805913742,7.8139934791502));
#11142=CARTESIAN_POINT('Ctrl Pts',(-0.354152161259447,1.04824937041078,
7.83630306607929));
#11143=CARTESIAN_POINT('Ctrl Pts',(-0.774821505581955,0.776301631566783,
7.85677186261233));
#11144=CARTESIAN_POINT('Ctrl Pts',(-1.01364810108653,0.395754395150175,
7.87539596090851));
#11145=CARTESIAN_POINT('Ctrl Pts',(-1.08917134999908,-0.00205304235367609,
7.89216907011948));
#11146=CARTESIAN_POINT('Ctrl Pts',(-1.01353540633159,-0.399628518798629,
7.90895346821961));
#11147=CARTESIAN_POINT('Ctrl Pts',(-0.727131996125876,-0.858432305737684,
7.93134780330843));
#11148=CARTESIAN_POINT('Ctrl Pts',(-0.0863637973312472,-1.16829644414184,
7.95936473371975));
#11149=CARTESIAN_POINT('Ctrl Pts',(0.732678237418673,-0.915943411696203,
7.99302779994513));
#11150=CARTESIAN_POINT('Ctrl Pts',(1.16109954417639,-0.173577431070782,
8.02672930691054));
#11151=CARTESIAN_POINT('Ctrl Pts',(0.970648308118703,0.663040508180315,
8.06046758095857));
#11152=CARTESIAN_POINT('Ctrl Pts',(0.260283477478894,1.14757073863936,8.09424060232552));
#11153=CARTESIAN_POINT('Ctrl Pts',(-0.494518330344157,1.03279226984595,
8.12428848091482));
#11154=CARTESIAN_POINT('Ctrl Pts',(-0.95478161188669,0.581876430066912,
8.15060205079116));
#11155=CARTESIAN_POINT('Ctrl Pts',(-1.11772856826109,0.0548873179080656,
8.17316849900046));
#11156=CARTESIAN_POINT('Ctrl Pts',(-1.00819355033569,-0.486661028909071,
8.19574690136803));
#11157=CARTESIAN_POINT('Ctrl Pts',(-0.653258105050941,-0.910215074380895,
8.21833809577143));
#11158=CARTESIAN_POINT('Ctrl Pts',(-0.267209331026347,-1.06136783567525,
8.23528758547523));
#11159=CARTESIAN_POINT('Ctrl Pts',(0.000873105475631335,-1.07790421719274,
8.24659249433198));
#11160=CARTESIAN_POINT('Ctrl Pts',(0.179526465106109,-1.06678600021225,
8.25412966597351));
#11161=CARTESIAN_POINT('Ctrl Pts',(0.441661152994394,-1.00025121357308,
8.26543678412909));
#11162=CARTESIAN_POINT('Ctrl Pts',(0.74897005908796,-0.806537047527932,
8.2805156563327));
#11163=CARTESIAN_POINT('Ctrl Pts',(1.07539940103965,-0.367786484198072,
8.30314183095587));
#11164=CARTESIAN_POINT('Ctrl Pts',(1.13073755868417,0.348336730332993,8.33143620802701));
#11165=CARTESIAN_POINT('Ctrl Pts',(0.590404903092466,1.0253443836268,8.3654006862316));
#11166=CARTESIAN_POINT('Ctrl Pts',(-0.191896495262822,1.14202728535317,
8.39654847127686));
#11167=CARTESIAN_POINT('Ctrl Pts',(-0.803630405103391,0.802689596644375,
8.42487470313664));
#11168=CARTESIAN_POINT('Ctrl Pts',(-1.10777223118505,0.252867678305614,
8.45037283391805));
#11169=CARTESIAN_POINT('Ctrl Pts',(-1.07264929230278,-0.375831789681131,
8.47587587326063));
#11170=CARTESIAN_POINT('Ctrl Pts',(-0.775756370582944,-0.793138595001687,
8.49665696129285));
#11171=CARTESIAN_POINT('Ctrl Pts',(-0.370973206955298,-1.04054893447855,
8.51649811440533));
#11172=CARTESIAN_POINT('Ctrl Pts',(0.038369462981197,-1.11292368936976,
8.53350571642248));
#11173=CARTESIAN_POINT('Ctrl Pts',(0.47898976689409,-0.994340382144285,
8.55240171155723));
#11174=CARTESIAN_POINT('Ctrl Pts',(0.80923417022507,-0.750922678629335,
8.56941016515415));
#11175=CARTESIAN_POINT('Ctrl Pts',(1.0274182871984,-0.403326067555486,8.58641602817986));
#11176=CARTESIAN_POINT('Ctrl Pts',(1.11691118054261,0.0671129407531136,
8.60625737788999));
#11177=CARTESIAN_POINT('Ctrl Pts',(0.962508000998029,0.604452525770246,
8.62892861065794));
#11178=CARTESIAN_POINT('Ctrl Pts',(0.493205548534116,1.02369118998224,8.65443255406071));
#11179=CARTESIAN_POINT('Ctrl Pts',(-0.126835973873531,1.12902274781952,
8.67993208193622));
#11180=CARTESIAN_POINT('Ctrl Pts',(-0.707895425994039,0.888341330697344,
8.70542701256162));
#11181=CARTESIAN_POINT('Ctrl Pts',(-1.07169802862448,0.375537140185558,
8.73091586806527));
#11182=CARTESIAN_POINT('Ctrl Pts',(-1.10692322919911,-0.252055003610382,
8.75639778158459));
#11183=CARTESIAN_POINT('Ctrl Pts',(-0.802931792932112,-0.802016307091765,
8.7818716346359));
#11184=CARTESIAN_POINT('Ctrl Pts',(-0.253135892745948,-1.10583889227955,
8.80733643557024));
#11185=CARTESIAN_POINT('Ctrl Pts',(0.373787124048757,-1.07059371077824,
8.83279114625073));
#11186=CARTESIAN_POINT('Ctrl Pts',(0.885644972309457,-0.707362970666774,
8.85823476032552));
#11187=CARTESIAN_POINT('Ctrl Pts',(1.1256782624904,-0.127754861211958,8.88366627230367));
#11188=CARTESIAN_POINT('Ctrl Pts',(1.02061722935054,0.490400628571495,8.90908465879932));
#11189=CARTESIAN_POINT('Ctrl Pts',(0.602991135209833,0.957653872010445,
8.93448895110668));
#11190=CARTESIAN_POINT('Ctrl Pts',(0.00120859626939015,1.13099126811469,
8.95987805769087));
#11191=CARTESIAN_POINT('Ctrl Pts',(-0.600287978023236,0.957707910761615,
8.98525114960464));
#11192=CARTESIAN_POINT('Ctrl Pts',(-1.00136692422523,0.508544235532217,
9.00966765026286));
#11193=CARTESIAN_POINT('Ctrl Pts',(-1.11475583894706,-0.0541766995265247,
9.03312999675204));
#11194=CARTESIAN_POINT('Ctrl Pts',(-0.952788419669591,-0.580292773132626,
9.05564117304827));
#11195=CARTESIAN_POINT('Ctrl Pts',(-0.591528141422974,-0.932614863756553,
9.07626128741052));
#11196=CARTESIAN_POINT('Ctrl Pts',(-0.164923344909653,-1.0810596235015,
9.0949942575564));
#11197=CARTESIAN_POINT('Ctrl Pts',(0.377658114142277,-1.06225637331858,
9.11746360413473));
#11198=CARTESIAN_POINT('Ctrl Pts',(0.848868791300341,-0.74246439931946,
9.13990987964604));
#11199=CARTESIAN_POINT('Ctrl Pts',(1.06344806548654,-0.244595576832108,
9.162338498867));
#11200=CARTESIAN_POINT('Ctrl Pts',(1.08562630996489,0.295649655289467,9.18475421262983));
#11201=CARTESIAN_POINT('Ctrl Pts',(0.730193182157616,0.912995733937815,
9.21274171873496));
#11202=CARTESIAN_POINT('Ctrl Pts',(0.0507146947130891,1.12120769041665,
9.24069241304767));
#11203=CARTESIAN_POINT('Ctrl Pts',(-0.469908160478353,0.98001973592613,
9.26303328476729));
#11204=CARTESIAN_POINT('Ctrl Pts',(-0.831281954576518,0.714080478677811,
9.28163790668312));
#11205=CARTESIAN_POINT('Ctrl Pts',(-1.0707247835365,0.274656717484436,9.30208197073574));
#11206=CARTESIAN_POINT('Ctrl Pts',(-1.07026628651612,-0.270334760718956,
9.32436700779422));
#11207=CARTESIAN_POINT('Ctrl Pts',(-0.81012944245468,-0.748778183184174,
9.34662760904691));
#11208=CARTESIAN_POINT('Ctrl Pts',(-0.352913623587519,-1.04349781871771,
9.36886459486743));
#11209=CARTESIAN_POINT('Ctrl Pts',(0.18892490073276,-1.08440077143083,9.39108033469003));
#11210=CARTESIAN_POINT('Ctrl Pts',(0.565010389578148,-0.914360468661282,
9.40794963584902));
#11211=CARTESIAN_POINT('Ctrl Pts',(0.767035294725711,-0.728425442708479,
9.41949991154068));
#11212=CARTESIAN_POINT('Ctrl Pts',(0.892355216546134,-0.575710200559469,
9.42781320640248));
#11213=CARTESIAN_POINT('Ctrl Pts',(1.05269478111425,-0.266393255154064,
9.44235418619472));
#11214=CARTESIAN_POINT('Ctrl Pts',(1.07555876507525,0.142080540702115,9.45895154635578));
#11215=CARTESIAN_POINT('Ctrl Pts',(0.933282910553863,0.513021814758867,
9.47553758890735));
#11216=CARTESIAN_POINT('Ctrl Pts',(0.695081061939374,0.830497822734072,
9.49211211559699));
#11217=CARTESIAN_POINT('Ctrl Pts',(0.248476724545638,1.07754915938558,9.51280614214995));
#11218=CARTESIAN_POINT('Ctrl Pts',(-0.362433114682866,1.04304224887823,
9.53760669954168));
#11219=CARTESIAN_POINT('Ctrl Pts',(-0.860534362744572,0.689473898600431,
9.56237202551932));
#11220=CARTESIAN_POINT('Ctrl Pts',(-1.09388928914477,0.125810273797895,
9.58710240698908));
#11221=CARTESIAN_POINT('Ctrl Pts',(-0.991713095702174,-0.474700208975981,
9.61179677753925));
#11222=CARTESIAN_POINT('Ctrl Pts',(-0.586315730889703,-0.928151038584933,
9.63645472421636));
#11223=CARTESIAN_POINT('Ctrl Pts',(-0.00268034821758927,-1.09615308592063,
9.66107559259117));
#11224=CARTESIAN_POINT('Ctrl Pts',(0.579985073663781,-0.928151554047772,
9.68565886740576));
#11225=CARTESIAN_POINT('Ctrl Pts',(0.983331340832418,-0.476604367726687,
9.71020401270546));
#11226=CARTESIAN_POINT('Ctrl Pts',(1.08445410902017,0.119383118454789,9.73471053368719));
#11227=CARTESIAN_POINT('Ctrl Pts',(0.85335961648174,0.676927075373189,9.75917795165438));
#11228=CARTESIAN_POINT('Ctrl Pts',(0.361848605557405,1.02549620846588,9.78360581484665));
#11229=CARTESIAN_POINT('Ctrl Pts',(-0.238792954238506,1.05907901718415,
9.80799368150402));
#11230=CARTESIAN_POINT('Ctrl Pts',(-0.764369402329827,0.768436104225106,
9.83234115979546));
#11231=CARTESIAN_POINT('Ctrl Pts',(-1.05427545134513,0.243589360885239,
9.85664781917723));
#11232=CARTESIAN_POINT('Ctrl Pts',(-1.02057935151888,-0.354025448888461,
9.88091336937157));
#11233=CARTESIAN_POINT('Ctrl Pts',(-0.674705848488251,-0.841316796753126,
9.90513727965942));
#11234=CARTESIAN_POINT('Ctrl Pts',(-0.123577927191511,-1.06944251069366,
9.92931960214379));
#11235=CARTESIAN_POINT('Ctrl Pts',(0.46338865969666,-0.969738708423244,
9.95345913840996));
#11236=CARTESIAN_POINT('Ctrl Pts',(0.906472097123054,-0.573379692131889,
9.97755753026823));
#11237=CARTESIAN_POINT('Ctrl Pts',(1.01577492904176,-0.193792191488556,
9.99359268772338));
#11238=CARTESIAN_POINT('Ctrl Pts',(1.01580058362196,-0.00322343436719488,
10.0016061503604));
#11239=CARTESIAN_POINT('Ctrl Pts',(0.999999575810999,0.00315098358513781,
7.20006622055264));
#11240=CARTESIAN_POINT('Ctrl Pts',(0.999974319608277,0.190760468856422,
7.20795524501636));
#11241=CARTESIAN_POINT('Ctrl Pts',(0.892344234443071,0.564401735476683,
7.22374165130483));
#11242=CARTESIAN_POINT('Ctrl Pts',(0.456170863303355,0.954569139239392,
7.24746551842362));
#11243=CARTESIAN_POINT('Ctrl Pts',(-0.121643296695006,1.0527111229517,7.27123039275792));
#11244=CARTESIAN_POINT('Ctrl Pts',(-0.664174499114347,0.828146653873478,
7.29503750827097));
#11245=CARTESIAN_POINT('Ctrl Pts',(-1.00466229107333,0.348451955041142,
7.31888617441183));
#11246=CARTESIAN_POINT('Ctrl Pts',(-1.03783821085617,-0.239862803165599,
7.34277653444097));
#11247=CARTESIAN_POINT('Ctrl Pts',(-0.752436914310739,-0.756562482852077,
7.36670833282365));
#11248=CARTESIAN_POINT('Ctrl Pts',(-0.234997931414651,-1.04270891419437,
7.39068146490982));
#11249=CARTESIAN_POINT('Ctrl Pts',(0.356377432582172,-1.00964746384867,
7.41469572763747));
#11250=CARTESIAN_POINT('Ctrl Pts',(0.840341677037224,-0.666437865062604,
7.43875093208249));
#11251=CARTESIAN_POINT('Ctrl Pts',(1.06790358406505,-0.117422164195028,
7.4628468515188));
#11252=CARTESIAN_POINT('Ctrl Pts',(0.968336509361683,0.469494166098508,
7.48698324256581));
#11253=CARTESIAN_POINT('Ctrl Pts',(0.571081336399399,0.914217869413367,
7.51115983904362));
#11254=CARTESIAN_POINT('Ctrl Pts',(-0.00276942901145937,1.07968430615977,
7.53537635143244));
#11255=CARTESIAN_POINT('Ctrl Pts',(-0.577781503135752,0.914223804149117,
7.55963247041146));
#11256=CARTESIAN_POINT('Ctrl Pts',(-0.962145622562424,0.483976677731404,
7.58302803095162));
#11257=CARTESIAN_POINT('Ctrl Pts',(-1.07125753086067,-0.0562794445165808,
7.60555779623404));
#11258=CARTESIAN_POINT('Ctrl Pts',(-0.915194862614763,-0.562561634031091,
7.6272168563822));
#11259=CARTESIAN_POINT('Ctrl Pts',(-0.53551487530705,-0.932963762094015,
7.64890612590553));
#11260=CARTESIAN_POINT('Ctrl Pts',(-0.024035065806305,-1.07736876663697,
7.67062531437742));
#11261=CARTESIAN_POINT('Ctrl Pts',(0.494146757015346,-0.958466814289234,
7.69237411680017));
#11262=CARTESIAN_POINT('Ctrl Pts',(0.961479539986573,-0.548279772601945,
7.71778190065853));
#11263=CARTESIAN_POINT('Ctrl Pts',(1.12756301652098,0.172482400610549,7.74686765103336));
#11264=CARTESIAN_POINT('Ctrl Pts',(0.75611713355168,0.813684959589575,7.77601030696451));
#11265=CARTESIAN_POINT('Ctrl Pts',(0.185875815215743,1.06965010757807,7.80155082448588));
#11266=CARTESIAN_POINT('Ctrl Pts',(-0.348517058347165,1.02984652160674,
7.82347022110603));
#11267=CARTESIAN_POINT('Ctrl Pts',(-0.761949296282463,0.762592777124389,
7.84358787235736));
#11268=CARTESIAN_POINT('Ctrl Pts',(-0.996722963062006,0.388518849169714,
7.86189613571743));
#11269=CARTESIAN_POINT('Ctrl Pts',(-1.07098690831041,-0.00260829917091459,
7.87838843437341));
#11270=CARTESIAN_POINT('Ctrl Pts',(-0.99661183226746,-0.393594984460838,
7.894895410549));
#11271=CARTESIAN_POINT('Ctrl Pts',(-0.714908576434247,-0.844892296878379,
7.9169240469514));
#11272=CARTESIAN_POINT('Ctrl Pts',(-0.084422651145012,-1.14985023564212,
7.94449562780488));
#11273=CARTESIAN_POINT('Ctrl Pts',(0.721887320494981,-0.901498071462995,
7.97763725360595));
#11274=CARTESIAN_POINT('Ctrl Pts',(1.14390600676876,-0.170383526932712,
8.01083302661308));
#11275=CARTESIAN_POINT('Ctrl Pts',(0.956311918053777,0.65401391794098,8.04408130906187));
#11276=CARTESIAN_POINT('Ctrl Pts',(0.25602906697655,1.13176193513965,8.07738040653961));
#11277=CARTESIAN_POINT('Ctrl Pts',(-0.488510543500641,1.01860423556296,
8.10702323570327));
#11278=CARTESIAN_POINT('Ctrl Pts',(-0.942716248260153,0.573655629467007,
8.13299136011509));
#11279=CARTESIAN_POINT('Ctrl Pts',(-1.10358636285334,0.0534364176198665,
8.15527022722507));
#11280=CARTESIAN_POINT('Ctrl Pts',(-0.99543872479676,-0.481361877750802,
8.17756901902506));
#11281=CARTESIAN_POINT('Ctrl Pts',(-0.644826641417894,-0.899786909633448,
8.1998871769012));
#11282=CARTESIAN_POINT('Ctrl Pts',(-0.263312902512338,-1.04918995788175,
8.21663989380025));
#11283=CARTESIAN_POINT('Ctrl Pts',(0.00166665731618679,-1.0655343402046,
8.22781406534667));
#11284=CARTESIAN_POINT('Ctrl Pts',(0.178270288589001,-1.05454413855026,
8.23526501957515));
#11285=CARTESIAN_POINT('Ctrl Pts',(0.437439999691742,-0.98876491629653,
8.24644481283225));
#11286=CARTESIAN_POINT('Ctrl Pts',(0.741357296669408,-0.797196125183601,
8.26135855011107));
#11287=CARTESIAN_POINT('Ctrl Pts',(1.06427742047819,-0.363196133741635,
8.28374205636937));
#11288=CARTESIAN_POINT('Ctrl Pts',(1.1191132547847,0.345488423812591,8.31174498186711));
#11289=CARTESIAN_POINT('Ctrl Pts',(0.584140656179565,1.01596202851522,8.34538413710338));
#11290=CARTESIAN_POINT('Ctrl Pts',(-0.19096844855633,1.13165287559935,8.37625078730322));
#11291=CARTESIAN_POINT('Ctrl Pts',(-0.797411359462935,0.795301993540907,
8.40433431031039));
#11292=CARTESIAN_POINT('Ctrl Pts',(-1.0990783559073,0.250015446968417,8.4296262708737));
#11293=CARTESIAN_POINT('Ctrl Pts',(-1.06426569125542,-0.373802040240765,
8.45493410201599));
#11294=CARTESIAN_POINT('Ctrl Pts',(-0.769553388901587,-0.788092512102153,
8.47556748693345));
#11295=CARTESIAN_POINT('Ctrl Pts',(-0.367608264833719,-1.03377453912702,
8.49527086803642));
#11296=CARTESIAN_POINT('Ctrl Pts',(0.0389894662197936,-1.10568483145998,
8.51216552927169));
#11297=CARTESIAN_POINT('Ctrl Pts',(0.476842798425807,-0.987859734068039,
8.53094473644388));
#11298=CARTESIAN_POINT('Ctrl Pts',(0.805101130351003,-0.7459169684144,8.54785141982868));
#11299=CARTESIAN_POINT('Ctrl Pts',(1.02206224073455,-0.400294829517718,
8.56476322077897));
#11300=CARTESIAN_POINT('Ctrl Pts',(1.11108597940432,0.0676090739442989,
8.58449929513004));
#11301=CARTESIAN_POINT('Ctrl Pts',(0.957486327179168,0.602305552598091,
8.60706239241156));
#11302=CARTESIAN_POINT('Ctrl Pts',(0.490319176226327,1.0196961225561,8.63245514939238));
#11303=CARTESIAN_POINT('Ctrl Pts',(-0.127227772869885,1.12465246691674,
8.65785621578684));
#11304=CARTESIAN_POINT('Ctrl Pts',(-0.706252354762176,0.884861784560879,
8.6832646175365));
#11305=CARTESIAN_POINT('Ctrl Pts',(-1.06898139570907,0.373646110671472,
8.70867937640931));
#11306=CARTESIAN_POINT('Ctrl Pts',(-1.10415883703196,-0.252336062683339,
8.73409951326223));
#11307=CARTESIAN_POINT('Ctrl Pts',(-0.800834752831557,-0.801177522527246,
8.75952404569165));
#11308=CARTESIAN_POINT('Ctrl Pts',(-0.251930241323733,-1.10455619700772,
8.78495198825788));
#11309=CARTESIAN_POINT('Ctrl Pts',(0.374309533721303,-1.06939244573458,
8.81038235029736));
#11310=CARTESIAN_POINT('Ctrl Pts',(0.88588373813812,-0.706416051605379,
8.83581414648952));
#11311=CARTESIAN_POINT('Ctrl Pts',(1.12593002076033,-0.126889341474946,
8.86124638643539));
#11312=CARTESIAN_POINT('Ctrl Pts',(1.02087104515559,0.491507891337351,8.88667807898767));
#11313=CARTESIAN_POINT('Ctrl Pts',(0.602911335681679,0.959196578831539,
8.91210823370906));
#11314=CARTESIAN_POINT('Ctrl Pts',(0.000316973456126708,1.13280882473463,
8.93753586563178));
#11315=CARTESIAN_POINT('Ctrl Pts',(-0.602311983560242,0.959240722445107,
8.9629599838141));
#11316=CARTESIAN_POINT('Ctrl Pts',(-1.00436822137552,0.509038661422071,
8.98743813657581));
#11317=CARTESIAN_POINT('Ctrl Pts',(-1.11811011681427,-0.0552669144060651,
9.01097002817133));
#11318=CARTESIAN_POINT('Ctrl Pts',(-0.955644771077333,-0.583087731975911,
9.03355562561233));
#11319=CARTESIAN_POINT('Ctrl Pts',(-0.593074356957321,-0.936728146430118,
9.0542538609391));
#11320=CARTESIAN_POINT('Ctrl Pts',(-0.164731041598437,-1.08578943530602,
9.07306578079699));
#11321=CARTESIAN_POINT('Ctrl Pts',(0.380219776536112,-1.06693040182505,
9.09563491033651));
#11322=CARTESIAN_POINT('Ctrl Pts',(0.853779549938941,-0.745621203287222,
9.11819570154211));
#11323=CARTESIAN_POINT('Ctrl Pts',(1.06953462325323,-0.245092836305948,
9.14074702398398));
#11324=CARTESIAN_POINT('Ctrl Pts',(1.09185195352203,0.298202592837182,9.16329164905568));
#11325=CARTESIAN_POINT('Ctrl Pts',(0.734297058725123,0.919425032182445,
9.19145918094331));
#11326=CARTESIAN_POINT('Ctrl Pts',(0.0501860572080287,1.12913650428628,
9.21960716991184));
#11327=CARTESIAN_POINT('Ctrl Pts',(-0.47422284767955,0.986938013732599,
9.24211273100823));
#11328=CARTESIAN_POINT('Ctrl Pts',(-0.83834294439581,0.718994011703782,
9.26085993499593));
#11329=CARTESIAN_POINT('Ctrl Pts',(-1.0797140885543,0.276058653254629,9.28147192866405));
#11330=CARTESIAN_POINT('Ctrl Pts',(-1.0792869722179,-0.273490761429736,
9.30394472055128));
#11331=CARTESIAN_POINT('Ctrl Pts',(-0.816874083948392,-0.756154521252702,
9.32640385818033));
#11332=CARTESIAN_POINT('Ctrl Pts',(-0.355458797527567,-1.05362205517351,
9.34884870640624));
#11333=CARTESIAN_POINT('Ctrl Pts',(0.191577194376755,-1.09493860698716,
9.37127864639074));
#11334=CARTESIAN_POINT('Ctrl Pts',(0.571484722667441,-0.923210767165354,
9.38832293897591));
#11335=CARTESIAN_POINT('Ctrl Pts',(0.775578610165073,-0.735373724461368,
9.39999172743641));
#11336=CARTESIAN_POINT('Ctrl Pts',(0.90219668945127,-0.581077610283799,
9.40839153478326));
#11337=CARTESIAN_POINT('Ctrl Pts',(1.06423218001646,-0.268505675241936,
9.42308663622534));
#11338=CARTESIAN_POINT('Ctrl Pts',(1.08737574685665,0.14445700622961,9.43987039483926));
#11339=CARTESIAN_POINT('Ctrl Pts',(0.943512119332504,0.519555849049532,
9.45664308969273));
#11340=CARTESIAN_POINT('Ctrl Pts',(0.702595952885493,0.840663912121189,
9.47340826939813));
#11341=CARTESIAN_POINT('Ctrl Pts',(0.250731034525726,1.09066378632527,9.49435038976507));
#11342=CARTESIAN_POINT('Ctrl Pts',(-0.367646366337481,1.05577469318307,
9.51945715090945));
#11343=CARTESIAN_POINT('Ctrl Pts',(-0.872073427555176,0.697769149747224,
9.54453931621249));
#11344=CARTESIAN_POINT('Ctrl Pts',(-1.10851395153864,0.126754498956172,
9.56959609551394));
#11345=CARTESIAN_POINT('Ctrl Pts',(-1.004997965557,-0.481859237919703,9.59462670660628));
#11346=CARTESIAN_POINT('Ctrl Pts',(-0.593994937248818,-0.94163509404227,
9.61963038098806));
#11347=CARTESIAN_POINT('Ctrl Pts',(-0.0020235655980388,-1.11207375119343,
9.6446063758667));
#11348=CARTESIAN_POINT('Ctrl Pts',(0.589215999041395,-0.941636436533483,
9.66955394755264));
#11349=CARTESIAN_POINT('Ctrl Pts',(0.99867475328867,-0.483298149068583,
9.69447238340543));
#11350=CARTESIAN_POINT('Ctrl Pts',(1.10139617547556,0.121906639873499,9.71936097538517));
#11351=CARTESIAN_POINT('Ctrl Pts',(0.866669607038716,0.688301956936916,
9.74421904187644));
#11352=CARTESIAN_POINT('Ctrl Pts',(0.367204775824758,1.0425526426198,9.76904590972932));
#11353=CARTESIAN_POINT('Ctrl Pts',(-0.243395435261487,1.07672488055471,
9.79384092765142));
#11354=CARTESIAN_POINT('Ctrl Pts',(-0.777888567237211,0.781186417289152,
9.81860345995005));
#11355=CARTESIAN_POINT('Ctrl Pts',(-1.07283036518199,0.247282943918733,
9.84333289822209));
#11356=CARTESIAN_POINT('Ctrl Pts',(-1.03856704754786,-0.360866232625645,
9.86802861303319));
#11357=CARTESIAN_POINT('Ctrl Pts',(-0.686501281653619,-0.856920605922548,
9.892690097101));
#11358=CARTESIAN_POINT('Ctrl Pts',(-0.125304938207573,-1.08924443021579,
9.91731661435472));
#11359=CARTESIAN_POINT('Ctrl Pts',(0.472593334675849,-0.987703022851267,
9.94190800522239));
#11360=CARTESIAN_POINT('Ctrl Pts',(0.924078607982629,-0.583894056083662,
9.9664628819065));
#11361=CARTESIAN_POINT('Ctrl Pts',(1.03553205098759,-0.196980695813872,
9.98281022139497));
#11362=CARTESIAN_POINT('Ctrl Pts',(1.03555819462295,-0.00277911247133682,
9.99097644525911));
#11363=CARTESIAN_POINT('',(0.999999575810999,0.00315098358513782,7.20006622055264));
#11364=CARTESIAN_POINT('Origin',(1.,0.,7.275));
#11365=CARTESIAN_POINT('',(1.03555819462295,-0.00277911247133681,9.99097644525911));
#11366=CARTESIAN_POINT('Ctrl Pts',(0.999999575810999,0.00315098358513781,
7.20006622055264));
#11367=CARTESIAN_POINT('Ctrl Pts',(0.999974319608277,0.190760468856422,
7.20795524501636));
#11368=CARTESIAN_POINT('Ctrl Pts',(0.892344234443071,0.564401735476683,
7.22374165130483));
#11369=CARTESIAN_POINT('Ctrl Pts',(0.456170863303355,0.954569139239392,
7.24746551842362));
#11370=CARTESIAN_POINT('Ctrl Pts',(-0.121643296695006,1.0527111229517,7.27123039275792));
#11371=CARTESIAN_POINT('Ctrl Pts',(-0.664174499114347,0.828146653873478,
7.29503750827097));
#11372=CARTESIAN_POINT('Ctrl Pts',(-1.00466229107333,0.348451955041142,
7.31888617441183));
#11373=CARTESIAN_POINT('Ctrl Pts',(-1.03783821085617,-0.239862803165599,
7.34277653444097));
#11374=CARTESIAN_POINT('Ctrl Pts',(-0.752436914310739,-0.756562482852077,
7.36670833282365));
#11375=CARTESIAN_POINT('Ctrl Pts',(-0.234997931414651,-1.04270891419437,
7.39068146490982));
#11376=CARTESIAN_POINT('Ctrl Pts',(0.356377432582172,-1.00964746384867,
7.41469572763747));
#11377=CARTESIAN_POINT('Ctrl Pts',(0.840341677037224,-0.666437865062604,
7.43875093208249));
#11378=CARTESIAN_POINT('Ctrl Pts',(1.06790358406505,-0.117422164195028,
7.4628468515188));
#11379=CARTESIAN_POINT('Ctrl Pts',(0.968336509361683,0.469494166098508,
7.48698324256581));
#11380=CARTESIAN_POINT('Ctrl Pts',(0.571081336399399,0.914217869413367,
7.51115983904362));
#11381=CARTESIAN_POINT('Ctrl Pts',(-0.00276942901145937,1.07968430615977,
7.53537635143244));
#11382=CARTESIAN_POINT('Ctrl Pts',(-0.577781503135752,0.914223804149117,
7.55963247041146));
#11383=CARTESIAN_POINT('Ctrl Pts',(-0.962145622562424,0.483976677731404,
7.58302803095162));
#11384=CARTESIAN_POINT('Ctrl Pts',(-1.07125753086067,-0.0562794445165808,
7.60555779623404));
#11385=CARTESIAN_POINT('Ctrl Pts',(-0.915194862614763,-0.562561634031091,
7.6272168563822));
#11386=CARTESIAN_POINT('Ctrl Pts',(-0.53551487530705,-0.932963762094015,
7.64890612590553));
#11387=CARTESIAN_POINT('Ctrl Pts',(-0.024035065806305,-1.07736876663697,
7.67062531437742));
#11388=CARTESIAN_POINT('Ctrl Pts',(0.494146757015346,-0.958466814289234,
7.69237411680017));
#11389=CARTESIAN_POINT('Ctrl Pts',(0.961479539986573,-0.548279772601945,
7.71778190065853));
#11390=CARTESIAN_POINT('Ctrl Pts',(1.12756301652098,0.172482400610549,7.74686765103336));
#11391=CARTESIAN_POINT('Ctrl Pts',(0.75611713355168,0.813684959589575,7.77601030696451));
#11392=CARTESIAN_POINT('Ctrl Pts',(0.185875815215743,1.06965010757807,7.80155082448588));
#11393=CARTESIAN_POINT('Ctrl Pts',(-0.348517058347165,1.02984652160674,
7.82347022110603));
#11394=CARTESIAN_POINT('Ctrl Pts',(-0.761949296282463,0.762592777124389,
7.84358787235736));
#11395=CARTESIAN_POINT('Ctrl Pts',(-0.996722963062006,0.388518849169714,
7.86189613571743));
#11396=CARTESIAN_POINT('Ctrl Pts',(-1.07098690831041,-0.00260829917091459,
7.87838843437341));
#11397=CARTESIAN_POINT('Ctrl Pts',(-0.99661183226746,-0.393594984460838,
7.894895410549));
#11398=CARTESIAN_POINT('Ctrl Pts',(-0.714908576434247,-0.844892296878379,
7.9169240469514));
#11399=CARTESIAN_POINT('Ctrl Pts',(-0.084422651145012,-1.14985023564212,
7.94449562780488));
#11400=CARTESIAN_POINT('Ctrl Pts',(0.721887320494981,-0.901498071462995,
7.97763725360595));
#11401=CARTESIAN_POINT('Ctrl Pts',(1.14390600676876,-0.170383526932712,
8.01083302661308));
#11402=CARTESIAN_POINT('Ctrl Pts',(0.956311918053777,0.65401391794098,8.04408130906187));
#11403=CARTESIAN_POINT('Ctrl Pts',(0.25602906697655,1.13176193513965,8.07738040653961));
#11404=CARTESIAN_POINT('Ctrl Pts',(-0.488510543500641,1.01860423556296,
8.10702323570327));
#11405=CARTESIAN_POINT('Ctrl Pts',(-0.942716248260153,0.573655629467007,
8.13299136011509));
#11406=CARTESIAN_POINT('Ctrl Pts',(-1.10358636285334,0.0534364176198665,
8.15527022722507));
#11407=CARTESIAN_POINT('Ctrl Pts',(-0.99543872479676,-0.481361877750802,
8.17756901902506));
#11408=CARTESIAN_POINT('Ctrl Pts',(-0.644826641417894,-0.899786909633448,
8.1998871769012));
#11409=CARTESIAN_POINT('Ctrl Pts',(-0.263312902512338,-1.04918995788175,
8.21663989380025));
#11410=CARTESIAN_POINT('Ctrl Pts',(0.00166665731618679,-1.0655343402046,
8.22781406534667));
#11411=CARTESIAN_POINT('Ctrl Pts',(0.178270288589001,-1.05454413855026,
8.23526501957515));
#11412=CARTESIAN_POINT('Ctrl Pts',(0.437439999691742,-0.98876491629653,
8.24644481283225));
#11413=CARTESIAN_POINT('Ctrl Pts',(0.741357296669408,-0.797196125183601,
8.26135855011107));
#11414=CARTESIAN_POINT('Ctrl Pts',(1.06427742047819,-0.363196133741635,
8.28374205636937));
#11415=CARTESIAN_POINT('Ctrl Pts',(1.1191132547847,0.345488423812591,8.31174498186711));
#11416=CARTESIAN_POINT('Ctrl Pts',(0.584140656179565,1.01596202851522,8.34538413710338));
#11417=CARTESIAN_POINT('Ctrl Pts',(-0.19096844855633,1.13165287559935,8.37625078730322));
#11418=CARTESIAN_POINT('Ctrl Pts',(-0.797411359462935,0.795301993540907,
8.40433431031039));
#11419=CARTESIAN_POINT('Ctrl Pts',(-1.0990783559073,0.250015446968417,8.4296262708737));
#11420=CARTESIAN_POINT('Ctrl Pts',(-1.06426569125542,-0.373802040240765,
8.45493410201599));
#11421=CARTESIAN_POINT('Ctrl Pts',(-0.769553388901587,-0.788092512102153,
8.47556748693345));
#11422=CARTESIAN_POINT('Ctrl Pts',(-0.367608264833719,-1.03377453912702,
8.49527086803642));
#11423=CARTESIAN_POINT('Ctrl Pts',(0.0389894662197936,-1.10568483145998,
8.51216552927169));
#11424=CARTESIAN_POINT('Ctrl Pts',(0.476842798425807,-0.987859734068039,
8.53094473644388));
#11425=CARTESIAN_POINT('Ctrl Pts',(0.805101130351003,-0.7459169684144,8.54785141982868));
#11426=CARTESIAN_POINT('Ctrl Pts',(1.02206224073455,-0.400294829517718,
8.56476322077897));
#11427=CARTESIAN_POINT('Ctrl Pts',(1.11108597940432,0.0676090739442989,
8.58449929513004));
#11428=CARTESIAN_POINT('Ctrl Pts',(0.957486327179168,0.602305552598091,
8.60706239241156));
#11429=CARTESIAN_POINT('Ctrl Pts',(0.490319176226327,1.0196961225561,8.63245514939238));
#11430=CARTESIAN_POINT('Ctrl Pts',(-0.127227772869885,1.12465246691674,
8.65785621578684));
#11431=CARTESIAN_POINT('Ctrl Pts',(-0.706252354762176,0.884861784560879,
8.6832646175365));
#11432=CARTESIAN_POINT('Ctrl Pts',(-1.06898139570907,0.373646110671472,
8.70867937640931));
#11433=CARTESIAN_POINT('Ctrl Pts',(-1.10415883703196,-0.252336062683339,
8.73409951326223));
#11434=CARTESIAN_POINT('Ctrl Pts',(-0.800834752831557,-0.801177522527246,
8.75952404569165));
#11435=CARTESIAN_POINT('Ctrl Pts',(-0.251930241323733,-1.10455619700772,
8.78495198825788));
#11436=CARTESIAN_POINT('Ctrl Pts',(0.374309533721303,-1.06939244573458,
8.81038235029736));
#11437=CARTESIAN_POINT('Ctrl Pts',(0.88588373813812,-0.706416051605379,
8.83581414648952));
#11438=CARTESIAN_POINT('Ctrl Pts',(1.12593002076033,-0.126889341474946,
8.86124638643539));
#11439=CARTESIAN_POINT('Ctrl Pts',(1.02087104515559,0.491507891337351,8.88667807898767));
#11440=CARTESIAN_POINT('Ctrl Pts',(0.602911335681679,0.959196578831539,
8.91210823370906));
#11441=CARTESIAN_POINT('Ctrl Pts',(0.000316973456126708,1.13280882473463,
8.93753586563178));
#11442=CARTESIAN_POINT('Ctrl Pts',(-0.602311983560242,0.959240722445107,
8.9629599838141));
#11443=CARTESIAN_POINT('Ctrl Pts',(-1.00436822137552,0.509038661422071,
8.98743813657581));
#11444=CARTESIAN_POINT('Ctrl Pts',(-1.11811011681427,-0.0552669144060651,
9.01097002817133));
#11445=CARTESIAN_POINT('Ctrl Pts',(-0.955644771077333,-0.583087731975911,
9.03355562561233));
#11446=CARTESIAN_POINT('Ctrl Pts',(-0.593074356957321,-0.936728146430118,
9.0542538609391));
#11447=CARTESIAN_POINT('Ctrl Pts',(-0.164731041598437,-1.08578943530602,
9.07306578079699));
#11448=CARTESIAN_POINT('Ctrl Pts',(0.380219776536112,-1.06693040182505,
9.09563491033651));
#11449=CARTESIAN_POINT('Ctrl Pts',(0.853779549938941,-0.745621203287222,
9.11819570154211));
#11450=CARTESIAN_POINT('Ctrl Pts',(1.06953462325323,-0.245092836305948,
9.14074702398398));
#11451=CARTESIAN_POINT('Ctrl Pts',(1.09185195352203,0.298202592837182,9.16329164905568));
#11452=CARTESIAN_POINT('Ctrl Pts',(0.734297058725123,0.919425032182445,
9.19145918094331));
#11453=CARTESIAN_POINT('Ctrl Pts',(0.0501860572080287,1.12913650428628,
9.21960716991184));
#11454=CARTESIAN_POINT('Ctrl Pts',(-0.47422284767955,0.986938013732599,
9.24211273100823));
#11455=CARTESIAN_POINT('Ctrl Pts',(-0.83834294439581,0.718994011703782,
9.26085993499593));
#11456=CARTESIAN_POINT('Ctrl Pts',(-1.0797140885543,0.276058653254629,9.28147192866405));
#11457=CARTESIAN_POINT('Ctrl Pts',(-1.0792869722179,-0.273490761429736,
9.30394472055128));
#11458=CARTESIAN_POINT('Ctrl Pts',(-0.816874083948392,-0.756154521252702,
9.32640385818033));
#11459=CARTESIAN_POINT('Ctrl Pts',(-0.355458797527567,-1.05362205517351,
9.34884870640624));
#11460=CARTESIAN_POINT('Ctrl Pts',(0.191577194376755,-1.09493860698716,
9.37127864639074));
#11461=CARTESIAN_POINT('Ctrl Pts',(0.571484722667441,-0.923210767165354,
9.38832293897591));
#11462=CARTESIAN_POINT('Ctrl Pts',(0.775578610165073,-0.735373724461368,
9.39999172743641));
#11463=CARTESIAN_POINT('Ctrl Pts',(0.90219668945127,-0.581077610283799,
9.40839153478326));
#11464=CARTESIAN_POINT('Ctrl Pts',(1.06423218001646,-0.268505675241936,
9.42308663622534));
#11465=CARTESIAN_POINT('Ctrl Pts',(1.08737574685665,0.14445700622961,9.43987039483926));
#11466=CARTESIAN_POINT('Ctrl Pts',(0.943512119332504,0.519555849049532,
9.45664308969273));
#11467=CARTESIAN_POINT('Ctrl Pts',(0.702595952885493,0.840663912121189,
9.47340826939813));
#11468=CARTESIAN_POINT('Ctrl Pts',(0.250731034525726,1.09066378632527,9.49435038976507));
#11469=CARTESIAN_POINT('Ctrl Pts',(-0.367646366337481,1.05577469318307,
9.51945715090945));
#11470=CARTESIAN_POINT('Ctrl Pts',(-0.872073427555176,0.697769149747224,
9.54453931621249));
#11471=CARTESIAN_POINT('Ctrl Pts',(-1.10851395153864,0.126754498956172,
9.56959609551394));
#11472=CARTESIAN_POINT('Ctrl Pts',(-1.004997965557,-0.481859237919703,9.59462670660628));
#11473=CARTESIAN_POINT('Ctrl Pts',(-0.593994937248818,-0.94163509404227,
9.61963038098806));
#11474=CARTESIAN_POINT('Ctrl Pts',(-0.0020235655980388,-1.11207375119343,
9.6446063758667));
#11475=CARTESIAN_POINT('Ctrl Pts',(0.589215999041395,-0.941636436533483,
9.66955394755264));
#11476=CARTESIAN_POINT('Ctrl Pts',(0.99867475328867,-0.483298149068583,
9.69447238340543));
#11477=CARTESIAN_POINT('Ctrl Pts',(1.10139617547556,0.121906639873499,9.71936097538517));
#11478=CARTESIAN_POINT('Ctrl Pts',(0.866669607038716,0.688301956936916,
9.74421904187644));
#11479=CARTESIAN_POINT('Ctrl Pts',(0.367204775824758,1.0425526426198,9.76904590972932));
#11480=CARTESIAN_POINT('Ctrl Pts',(-0.243395435261487,1.07672488055471,
9.79384092765142));
#11481=CARTESIAN_POINT('Ctrl Pts',(-0.777888567237211,0.781186417289152,
9.81860345995005));
#11482=CARTESIAN_POINT('Ctrl Pts',(-1.07283036518199,0.247282943918733,
9.84333289822209));
#11483=CARTESIAN_POINT('Ctrl Pts',(-1.03856704754786,-0.360866232625645,
9.86802861303319));
#11484=CARTESIAN_POINT('Ctrl Pts',(-0.686501281653619,-0.856920605922548,
9.892690097101));
#11485=CARTESIAN_POINT('Ctrl Pts',(-0.125304938207573,-1.08924443021579,
9.91731661435472));
#11486=CARTESIAN_POINT('Ctrl Pts',(0.472593334675849,-0.987703022851267,
9.94190800522239));
#11487=CARTESIAN_POINT('Ctrl Pts',(0.924078607982629,-0.583894056083662,
9.9664628819065));
#11488=CARTESIAN_POINT('Ctrl Pts',(1.03553205098759,-0.196980695813872,
9.98281022139497));
#11489=CARTESIAN_POINT('Ctrl Pts',(1.03555819462295,-0.00277911247133682,
9.99097644525911));
#11490=CARTESIAN_POINT('Origin',(1.,-2.33146835171283E-15,9.925));
#11491=CARTESIAN_POINT('Origin',(1.,-2.33146835171283E-15,9.925));
#11492=CARTESIAN_POINT('Origin',(1.,0.,7.275));
#12824=UNCERTAINTY_MEASURE_WITH_UNIT(LENGTH_MEASURE(0.001),#12897,
'DISTANCE_ACCURACY_VALUE',
'Maximum model space distance between geometric entities at asserted c
onnectivities');
#12853=UNCERTAINTY_MEASURE_WITH_UNIT(LENGTH_MEASURE(0.001),#12897,
'DISTANCE_ACCURACY_VALUE',
'Maximum model space distance between geometric entities at asserted c
onnectivities');
#12867=(
GEOMETRIC_REPRESENTATION_CONTEXT(3)
GLOBAL_UNCERTAINTY_ASSIGNED_CONTEXT((#12824))
GLOBAL_UNIT_ASSIGNED_CONTEXT((#12897,#12899,#12900))
REPRESENTATION_CONTEXT('','3D')
);
#12896=(
GEOMETRIC_REPRESENTATION_CONTEXT(3)
GLOBAL_UNCERTAINTY_ASSIGNED_CONTEXT((#12853))
GLOBAL_UNIT_ASSIGNED_CONTEXT((#12897,#12899,#12900))
REPRESENTATION_CONTEXT('','3D')
);
#12897=(
LENGTH_UNIT()
NAMED_UNIT(*)
SI_UNIT(.CENTI.,.METRE.)
);
#12899=(
NAMED_UNIT(*)
PLANE_ANGLE_UNIT()
SI_UNIT($,.RADIAN.)
);
#12900=(
NAMED_UNIT(*)
SI_UNIT($,.STERADIAN.)
SOLID_ANGLE_UNIT()
);
#12914=SHAPE_DEFINITION_REPRESENTATION(#12956,#13067);
#12956=PRODUCT_DEFINITION_SHAPE('',$,#13110);
#13067=SHAPE_REPRESENTATION('',(#6909),#12867);
#13096=PRODUCT_DEFINITION_CONTEXT('part definition',#13224,'design');
#13110=PRODUCT_DEFINITION('Installed return spring',
'Installed return spring',#13152,#13096);
#13152=PRODUCT_DEFINITION_FORMATION('',$,#13239);
#13224=APPLICATION_CONTEXT(
'Core Data for Automotive Mechanical Design Process');
#13225=PRODUCT_CONTEXT('part definition',#13224,'mechanical');
#13239=PRODUCT('Installed return spring','Installed return spring',
'Installed return spring',(#13225));
#13324=COLOUR_RGB('Grey',0.48,0.52,0.57);
#13325=FILL_AREA_STYLE_COLOUR('',#13324);
#13326=FILL_AREA_STYLE('',(#13325));
#13327=SURFACE_STYLE_FILL_AREA(#13326);
#13328=SURFACE_SIDE_STYLE('',(#13327));
#13329=SURFACE_STYLE_USAGE(.BOTH.,#13328);
#13330=PRESENTATION_STYLE_ASSIGNMENT((#13329));
ENDSEC;
END-ISO-10303-21;
